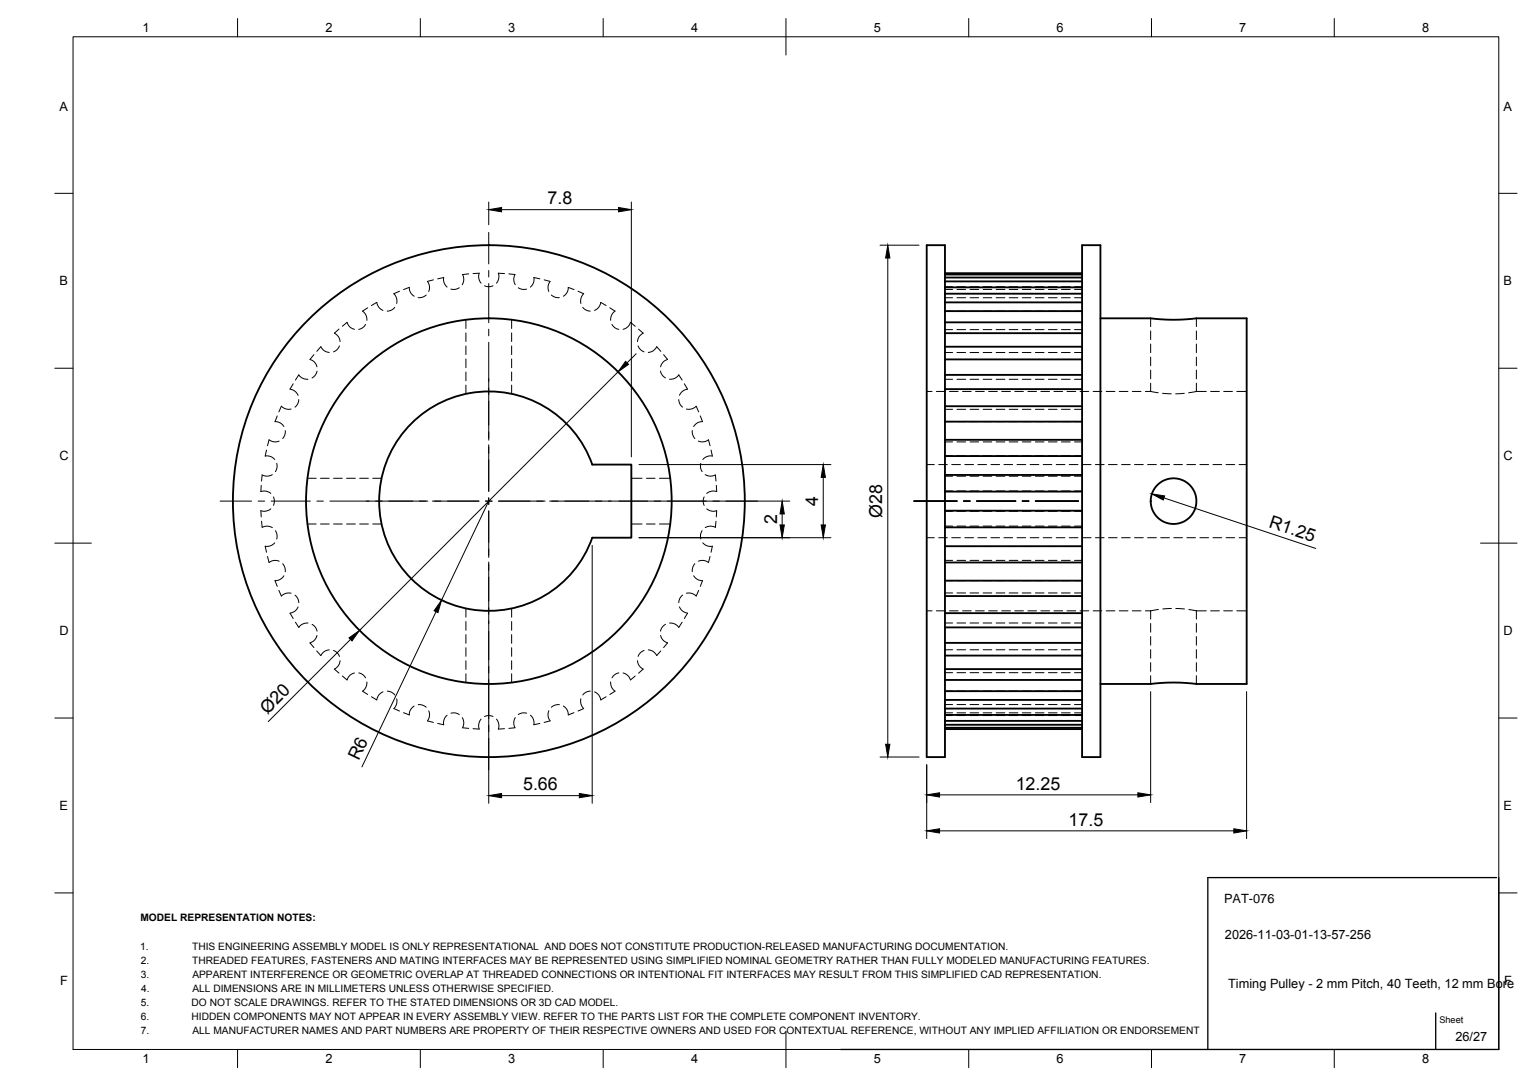
ISO-10303-21;
HEADER;
/* Generated by software containing ST-Developer
 * from STEP Tools, Inc. (www.steptools.com) 
 */

FILE_DESCRIPTION(
/* description */ ('Overhung pulley bearing cartridge'),
/* implementation_level */ '2;1');

FILE_NAME(
/* name */ 'Timing Pulley - 2 mm Pitch, 40 Teeth, 12 mm Bore.step',
/* time_stamp */ '2026-10-28T03:22:33-07:00',
/* author */ (''),
/* organization */ (''),
/* preprocessor_version */ 'ST-DEVELOPER v20.2',
/* originating_system */ 'Autodesk Translation Framework v15.17.0.0',
/* authorisation */ '');

FILE_SCHEMA (('AUTOMOTIVE_DESIGN { 1 0 10303 214 3 1 1 }'));
ENDSEC;

DATA;
#10=MECHANICAL_DESIGN_GEOMETRIC_PRESENTATION_REPRESENTATION('',(#310),#10963);
#189=B_SPLINE_CURVE_WITH_KNOTS('',3,(#10010,#10011,#10012,#10013,#10014,
#10015,#10016,#10017,#10018,#10019,#10020,#10021,#10022,#10023,#10024,#10025,
#10026,#10027),.UNSPECIFIED.,.F.,.F.,(4,2,2,2,2,2,2,2,4),(0.,0.0472365751919841,
0.0944731503839683,0.14170659898184,0.188940047579712,0.236173496177583,
0.283406944775455,0.330643519967439,0.377880095159423),.UNSPECIFIED.);
#190=B_SPLINE_CURVE_WITH_KNOTS('',3,(#10028,#10029,#10030,#10031,#10032,
#10033,#10034,#10035,#10036,#10037,#10038,#10039,#10040,#10041,#10042,#10043,
#10044,#10045),.UNSPECIFIED.,.F.,.F.,(4,2,2,2,2,2,2,2,4),(0.377880095159423,
0.425116670351408,0.472353245543392,0.519586694141263,0.566820142739135,
0.614053591337007,0.661287039934879,0.708523615126863,0.755760190318847),
 .UNSPECIFIED.);
#191=B_SPLINE_CURVE_WITH_KNOTS('',3,(#10048,#10049,#10050,#10051,#10052,
#10053,#10054,#10055,#10056,#10057,#10058,#10059,#10060,#10061,#10062,#10063,
#10064,#10065),.UNSPECIFIED.,.F.,.F.,(4,2,2,2,2,2,2,2,4),(0.,0.0472365751919841,
0.0944731503839682,0.14170659898184,0.188940047579712,0.236173496177583,
0.283406944775455,0.330643519967439,0.377880095159423),.UNSPECIFIED.);
#192=B_SPLINE_CURVE_WITH_KNOTS('',3,(#10066,#10067,#10068,#10069,#10070,
#10071,#10072,#10073,#10074,#10075,#10076,#10077,#10078,#10079,#10080,#10081,
#10082,#10083),.UNSPECIFIED.,.F.,.F.,(4,2,2,2,2,2,2,2,4),(0.377880095159423,
0.425116670351408,0.472353245543392,0.519586694141263,0.566820142739135,
0.614053591337007,0.661287039934879,0.708523615126863,0.755760190318847),
 .UNSPECIFIED.);
#193=B_SPLINE_CURVE_WITH_KNOTS('',3,(#10086,#10087,#10088,#10089,#10090,
#10091,#10092,#10093,#10094,#10095,#10096,#10097,#10098,#10099,#10100,#10101,
#10102,#10103),.UNSPECIFIED.,.F.,.F.,(4,2,2,2,2,2,2,2,4),(0.,0.0472365751919841,
0.0944731503839683,0.14170659898184,0.188940047579712,0.236173496177583,
0.283406944775455,0.330643519967439,0.377880095159423),.UNSPECIFIED.);
#194=B_SPLINE_CURVE_WITH_KNOTS('',3,(#10104,#10105,#10106,#10107,#10108,
#10109,#10110,#10111,#10112,#10113,#10114,#10115,#10116,#10117,#10118,#10119,
#10120,#10121),.UNSPECIFIED.,.F.,.F.,(4,2,2,2,2,2,2,2,4),(0.377880095159423,
0.425116670351408,0.472353245543392,0.519586694141263,0.566820142739135,
0.614053591337007,0.661287039934879,0.708523615126863,0.755760190318847),
 .UNSPECIFIED.);
#195=B_SPLINE_CURVE_WITH_KNOTS('',3,(#10125,#10126,#10127,#10128,#10129,
#10130,#10131,#10132,#10133,#10134),.UNSPECIFIED.,.F.,.F.,(4,2,2,2,4),(0.565665723963061,
0.61280433739166,0.659942950820258,0.70708195805217,0.754220965284082),
 .UNSPECIFIED.);
#196=B_SPLINE_CURVE_WITH_KNOTS('',3,(#10136,#10137,#10138,#10139,#10140,
#10141,#10142,#10143,#10144,#10145,#10146,#10147,#10148,#10149,#10150,#10151,
#10152,#10153),.UNSPECIFIED.,.F.,.F.,(4,2,2,2,2,2,2,2,4),(0.18855524132102,
0.235693854749619,0.282832468178217,0.329971475410129,0.377110482642041,
0.424249489873953,0.471388497105864,0.518527110534463,0.565665723963061),
 .UNSPECIFIED.);
#197=B_SPLINE_CURVE_WITH_KNOTS('',3,(#10154,#10155,#10156,#10157,#10158,
#10159,#10160,#10161,#10162,#10163),.UNSPECIFIED.,.F.,.F.,(4,2,2,2,4),(0.754220965284082,
0.801359972515993,0.848498979747905,0.895637593176504,0.942776206605102),
 .UNSPECIFIED.);
#198=B_SPLINE_CURVE_WITH_KNOTS('',3,(#10169,#10170,#10171,#10172,#10173,
#10174,#10175,#10176,#10177,#10178),.UNSPECIFIED.,.F.,.F.,(4,2,2,2,4),(0.565665723963061,
0.61280433739166,0.659942950820258,0.70708195805217,0.754220965284082),
 .UNSPECIFIED.);
#199=B_SPLINE_CURVE_WITH_KNOTS('',3,(#10180,#10181,#10182,#10183,#10184,
#10185,#10186,#10187,#10188,#10189,#10190,#10191,#10192,#10193,#10194,#10195,
#10196,#10197),.UNSPECIFIED.,.F.,.F.,(4,2,2,2,2,2,2,2,4),(0.18855524132102,
0.235693854749619,0.282832468178217,0.329971475410129,0.377110482642041,
0.424249489873953,0.471388497105864,0.518527110534463,0.565665723963061),
 .UNSPECIFIED.);
#200=B_SPLINE_CURVE_WITH_KNOTS('',3,(#10198,#10199,#10200,#10201,#10202,
#10203,#10204,#10205,#10206,#10207),.UNSPECIFIED.,.F.,.F.,(4,2,2,2,4),(0.754220965284082,
0.801359972515993,0.848498979747905,0.895637593176504,0.942776206605102),
 .UNSPECIFIED.);
#201=B_SPLINE_CURVE_WITH_KNOTS('',3,(#10217,#10218,#10219,#10220,#10221,
#10222,#10223,#10224,#10225,#10226,#10227,#10228,#10229,#10230,#10231,#10232,
#10233,#10234),.UNSPECIFIED.,.F.,.F.,(4,2,2,2,2,2,2,2,4),(0.18855524132102,
0.235693854749619,0.282832468178217,0.329971475410129,0.377110482642041,
0.424249489873953,0.471388497105864,0.518527110534463,0.565665723963061),
 .UNSPECIFIED.);
#202=B_SPLINE_CURVE_WITH_KNOTS('',3,(#10236,#10237,#10238,#10239,#10240,
#10241,#10242,#10243,#10244,#10245),.UNSPECIFIED.,.F.,.F.,(4,2,2,2,4),(0.565665723963061,
0.61280433739166,0.659942950820258,0.70708195805217,0.754220965284082),
 .UNSPECIFIED.);
#203=B_SPLINE_CURVE_WITH_KNOTS('',3,(#10246,#10247,#10248,#10249,#10250,
#10251,#10252,#10253,#10254,#10255),.UNSPECIFIED.,.F.,.F.,(4,2,2,2,4),(0.754220965284082,
0.801359972515993,0.848498979747905,0.895637593176504,0.942776206605102),
 .UNSPECIFIED.);
#204=B_SPLINE_CURVE_WITH_KNOTS('',3,(#10258,#10259,#10260,#10261,#10262,
#10263,#10264,#10265,#10266,#10267,#10268,#10269,#10270,#10271,#10272,#10273,
#10274,#10275),.UNSPECIFIED.,.F.,.F.,(4,2,2,2,2,2,2,2,4),(0.18855524132102,
0.235693854749619,0.282832468178217,0.329971475410129,0.377110482642041,
0.424249489873953,0.471388497105864,0.518527110534463,0.565665723963061),
 .UNSPECIFIED.);
#205=B_SPLINE_CURVE_WITH_KNOTS('',3,(#10277,#10278,#10279,#10280,#10281,
#10282,#10283,#10284,#10285,#10286),.UNSPECIFIED.,.F.,.F.,(4,2,2,2,4),(0.565665723963061,
0.61280433739166,0.659942950820258,0.70708195805217,0.754220965284082),
 .UNSPECIFIED.);
#206=B_SPLINE_CURVE_WITH_KNOTS('',3,(#10287,#10288,#10289,#10290,#10291,
#10292,#10293,#10294,#10295,#10296),.UNSPECIFIED.,.F.,.F.,(4,2,2,2,4),(0.754220965284082,
0.801359972515993,0.848498979747905,0.895637593176504,0.942776206605102),
 .UNSPECIFIED.);
#258=SHAPE_REPRESENTATION_RELATIONSHIP('SRR','None',#11080,#280);
#280=ADVANCED_BREP_SHAPE_REPRESENTATION('',(#338),#10960);
#310=STYLED_ITEM('',(#11246),#338);
#338=MANIFOLD_SOLID_BREP('Body1',#5679);
#421=FACE_BOUND('',#1199,.T.);
#422=FACE_BOUND('',#1202,.T.);
#423=FACE_BOUND('',#1204,.T.);
#424=FACE_BOUND('',#1205,.T.);
#425=FACE_BOUND('',#1206,.T.);
#426=FACE_BOUND('',#1210,.T.);
#427=FACE_BOUND('',#1211,.T.);
#428=FACE_BOUND('',#1212,.T.);
#429=FACE_BOUND('',#1216,.T.);
#430=FACE_BOUND('',#1218,.T.);
#431=FACE_BOUND('',#1221,.T.);
#432=FACE_BOUND('',#1223,.T.);
#550=PLANE('',#6385);
#551=PLANE('',#6386);
#552=PLANE('',#6388);
#553=PLANE('',#6389);
#554=PLANE('',#6401);
#555=PLANE('',#6402);
#556=PLANE('',#6486);
#557=PLANE('',#6487);
#788=FACE_OUTER_BOUND('',#1197,.T.);
#789=FACE_OUTER_BOUND('',#1198,.T.);
#790=FACE_OUTER_BOUND('',#1200,.T.);
#791=FACE_OUTER_BOUND('',#1201,.T.);
#792=FACE_OUTER_BOUND('',#1203,.T.);
#793=FACE_OUTER_BOUND('',#1207,.T.);
#794=FACE_OUTER_BOUND('',#1208,.T.);
#795=FACE_OUTER_BOUND('',#1209,.T.);
#796=FACE_OUTER_BOUND('',#1213,.T.);
#797=FACE_OUTER_BOUND('',#1214,.T.);
#798=FACE_OUTER_BOUND('',#1215,.T.);
#799=FACE_OUTER_BOUND('',#1217,.T.);
#800=FACE_OUTER_BOUND('',#1219,.T.);
#801=FACE_OUTER_BOUND('',#1220,.T.);
#802=FACE_OUTER_BOUND('',#1222,.T.);
#803=FACE_OUTER_BOUND('',#1224,.T.);
#804=FACE_OUTER_BOUND('',#1225,.T.);
#805=FACE_OUTER_BOUND('',#1226,.T.);
#806=FACE_OUTER_BOUND('',#1227,.T.);
#807=FACE_OUTER_BOUND('',#1228,.T.);
#808=FACE_OUTER_BOUND('',#1229,.T.);
#809=FACE_OUTER_BOUND('',#1230,.T.);
#810=FACE_OUTER_BOUND('',#1231,.T.);
#811=FACE_OUTER_BOUND('',#1232,.T.);
#812=FACE_OUTER_BOUND('',#1233,.T.);
#813=FACE_OUTER_BOUND('',#1234,.T.);
#814=FACE_OUTER_BOUND('',#1235,.T.);
#815=FACE_OUTER_BOUND('',#1236,.T.);
#816=FACE_OUTER_BOUND('',#1237,.T.);
#817=FACE_OUTER_BOUND('',#1238,.T.);
#818=FACE_OUTER_BOUND('',#1239,.T.);
#819=FACE_OUTER_BOUND('',#1240,.T.);
#820=FACE_OUTER_BOUND('',#1241,.T.);
#821=FACE_OUTER_BOUND('',#1242,.T.);
#822=FACE_OUTER_BOUND('',#1243,.T.);
#823=FACE_OUTER_BOUND('',#1244,.T.);
#824=FACE_OUTER_BOUND('',#1245,.T.);
#825=FACE_OUTER_BOUND('',#1246,.T.);
#826=FACE_OUTER_BOUND('',#1247,.T.);
#827=FACE_OUTER_BOUND('',#1248,.T.);
#828=FACE_OUTER_BOUND('',#1249,.T.);
#829=FACE_OUTER_BOUND('',#1250,.T.);
#830=FACE_OUTER_BOUND('',#1251,.T.);
#831=FACE_OUTER_BOUND('',#1252,.T.);
#832=FACE_OUTER_BOUND('',#1253,.T.);
#833=FACE_OUTER_BOUND('',#1254,.T.);
#834=FACE_OUTER_BOUND('',#1255,.T.);
#835=FACE_OUTER_BOUND('',#1256,.T.);
#836=FACE_OUTER_BOUND('',#1257,.T.);
#837=FACE_OUTER_BOUND('',#1258,.T.);
#838=FACE_OUTER_BOUND('',#1259,.T.);
#839=FACE_OUTER_BOUND('',#1260,.T.);
#840=FACE_OUTER_BOUND('',#1261,.T.);
#841=FACE_OUTER_BOUND('',#1262,.T.);
#842=FACE_OUTER_BOUND('',#1263,.T.);
#843=FACE_OUTER_BOUND('',#1264,.T.);
#844=FACE_OUTER_BOUND('',#1265,.T.);
#845=FACE_OUTER_BOUND('',#1266,.T.);
#846=FACE_OUTER_BOUND('',#1267,.T.);
#847=FACE_OUTER_BOUND('',#1268,.T.);
#848=FACE_OUTER_BOUND('',#1269,.T.);
#849=FACE_OUTER_BOUND('',#1270,.T.);
#850=FACE_OUTER_BOUND('',#1271,.T.);
#851=FACE_OUTER_BOUND('',#1272,.T.);
#852=FACE_OUTER_BOUND('',#1273,.T.);
#853=FACE_OUTER_BOUND('',#1274,.T.);
#854=FACE_OUTER_BOUND('',#1275,.T.);
#855=FACE_OUTER_BOUND('',#1276,.T.);
#856=FACE_OUTER_BOUND('',#1277,.T.);
#857=FACE_OUTER_BOUND('',#1278,.T.);
#858=FACE_OUTER_BOUND('',#1279,.T.);
#859=FACE_OUTER_BOUND('',#1280,.T.);
#860=FACE_OUTER_BOUND('',#1281,.T.);
#861=FACE_OUTER_BOUND('',#1282,.T.);
#862=FACE_OUTER_BOUND('',#1283,.T.);
#863=FACE_OUTER_BOUND('',#1284,.T.);
#864=FACE_OUTER_BOUND('',#1285,.T.);
#865=FACE_OUTER_BOUND('',#1286,.T.);
#866=FACE_OUTER_BOUND('',#1287,.T.);
#867=FACE_OUTER_BOUND('',#1288,.T.);
#868=FACE_OUTER_BOUND('',#1289,.T.);
#869=FACE_OUTER_BOUND('',#1290,.T.);
#870=FACE_OUTER_BOUND('',#1291,.T.);
#871=FACE_OUTER_BOUND('',#1292,.T.);
#872=FACE_OUTER_BOUND('',#1293,.T.);
#873=FACE_OUTER_BOUND('',#1294,.T.);
#874=FACE_OUTER_BOUND('',#1295,.T.);
#875=FACE_OUTER_BOUND('',#1296,.T.);
#876=FACE_OUTER_BOUND('',#1297,.T.);
#877=FACE_OUTER_BOUND('',#1298,.T.);
#878=FACE_OUTER_BOUND('',#1299,.T.);
#879=FACE_OUTER_BOUND('',#1300,.T.);
#880=FACE_OUTER_BOUND('',#1301,.T.);
#881=FACE_OUTER_BOUND('',#1302,.T.);
#882=FACE_OUTER_BOUND('',#1303,.T.);
#883=FACE_OUTER_BOUND('',#1304,.T.);
#1197=EDGE_LOOP('',(#4499,#4500,#4501,#4502));
#1198=EDGE_LOOP('',(#4503,#4504,#4505,#4506));
#1199=EDGE_LOOP('',(#4507));
#1200=EDGE_LOOP('',(#4508,#4509,#4510,#4511));
#1201=EDGE_LOOP('',(#4512));
#1202=EDGE_LOOP('',(#4513,#4514,#4515,#4516));
#1203=EDGE_LOOP('',(#4517,#4518,#4519,#4520));
#1204=EDGE_LOOP('',(#4521,#4522));
#1205=EDGE_LOOP('',(#4523,#4524));
#1206=EDGE_LOOP('',(#4525,#4526));
#1207=EDGE_LOOP('',(#4527,#4528,#4529,#4530,#4531,#4532,#4533));
#1208=EDGE_LOOP('',(#4534,#4535,#4536,#4537,#4538,#4539,#4540));
#1209=EDGE_LOOP('',(#4541,#4542,#4543,#4544,#4545,#4546,#4547,#4548,#4549));
#1210=EDGE_LOOP('',(#4550,#4551,#4552));
#1211=EDGE_LOOP('',(#4553,#4554,#4555));
#1212=EDGE_LOOP('',(#4556,#4557,#4558));
#1213=EDGE_LOOP('',(#4559,#4560,#4561,#4562,#4563,#4564));
#1214=EDGE_LOOP('',(#4565,#4566,#4567,#4568,#4569,#4570,#4571));
#1215=EDGE_LOOP('',(#4572));
#1216=EDGE_LOOP('',(#4573,#4574,#4575,#4576));
#1217=EDGE_LOOP('',(#4577));
#1218=EDGE_LOOP('',(#4578,#4579,#4580,#4581,#4582,#4583,#4584,#4585,#4586,
#4587,#4588,#4589,#4590,#4591,#4592,#4593,#4594,#4595,#4596,#4597,#4598,
#4599,#4600,#4601,#4602,#4603,#4604,#4605,#4606,#4607,#4608,#4609,#4610,
#4611,#4612,#4613,#4614,#4615,#4616,#4617,#4618,#4619,#4620,#4621,#4622,
#4623,#4624,#4625,#4626,#4627,#4628,#4629,#4630,#4631,#4632,#4633,#4634,
#4635,#4636,#4637,#4638,#4639,#4640,#4641,#4642,#4643,#4644,#4645,#4646,
#4647,#4648,#4649,#4650,#4651,#4652,#4653,#4654,#4655,#4656,#4657));
#1219=EDGE_LOOP('',(#4658,#4659,#4660,#4661));
#1220=EDGE_LOOP('',(#4662));
#1221=EDGE_LOOP('',(#4663));
#1222=EDGE_LOOP('',(#4664));
#1223=EDGE_LOOP('',(#4665,#4666,#4667,#4668,#4669,#4670,#4671,#4672,#4673,
#4674,#4675,#4676,#4677,#4678,#4679,#4680,#4681,#4682,#4683,#4684,#4685,
#4686,#4687,#4688,#4689,#4690,#4691,#4692,#4693,#4694,#4695,#4696,#4697,
#4698,#4699,#4700,#4701,#4702,#4703,#4704,#4705,#4706,#4707,#4708,#4709,
#4710,#4711,#4712,#4713,#4714,#4715,#4716,#4717,#4718,#4719,#4720,#4721,
#4722,#4723,#4724,#4725,#4726,#4727,#4728,#4729,#4730,#4731,#4732,#4733,
#4734,#4735,#4736,#4737,#4738,#4739,#4740,#4741,#4742,#4743,#4744));
#1224=EDGE_LOOP('',(#4745,#4746,#4747,#4748));
#1225=EDGE_LOOP('',(#4749,#4750,#4751,#4752));
#1226=EDGE_LOOP('',(#4753,#4754,#4755,#4756));
#1227=EDGE_LOOP('',(#4757,#4758,#4759,#4760));
#1228=EDGE_LOOP('',(#4761,#4762,#4763,#4764));
#1229=EDGE_LOOP('',(#4765,#4766,#4767,#4768));
#1230=EDGE_LOOP('',(#4769,#4770,#4771,#4772));
#1231=EDGE_LOOP('',(#4773,#4774,#4775,#4776));
#1232=EDGE_LOOP('',(#4777,#4778,#4779,#4780));
#1233=EDGE_LOOP('',(#4781,#4782,#4783,#4784));
#1234=EDGE_LOOP('',(#4785,#4786,#4787,#4788));
#1235=EDGE_LOOP('',(#4789,#4790,#4791,#4792));
#1236=EDGE_LOOP('',(#4793,#4794,#4795,#4796));
#1237=EDGE_LOOP('',(#4797,#4798,#4799,#4800));
#1238=EDGE_LOOP('',(#4801,#4802,#4803,#4804));
#1239=EDGE_LOOP('',(#4805,#4806,#4807,#4808));
#1240=EDGE_LOOP('',(#4809,#4810,#4811,#4812));
#1241=EDGE_LOOP('',(#4813,#4814,#4815,#4816));
#1242=EDGE_LOOP('',(#4817,#4818,#4819,#4820));
#1243=EDGE_LOOP('',(#4821,#4822,#4823,#4824));
#1244=EDGE_LOOP('',(#4825,#4826,#4827,#4828));
#1245=EDGE_LOOP('',(#4829,#4830,#4831,#4832));
#1246=EDGE_LOOP('',(#4833,#4834,#4835,#4836));
#1247=EDGE_LOOP('',(#4837,#4838,#4839,#4840));
#1248=EDGE_LOOP('',(#4841,#4842,#4843,#4844));
#1249=EDGE_LOOP('',(#4845,#4846,#4847,#4848));
#1250=EDGE_LOOP('',(#4849,#4850,#4851,#4852));
#1251=EDGE_LOOP('',(#4853,#4854,#4855,#4856));
#1252=EDGE_LOOP('',(#4857,#4858,#4859,#4860));
#1253=EDGE_LOOP('',(#4861,#4862,#4863,#4864));
#1254=EDGE_LOOP('',(#4865,#4866,#4867,#4868));
#1255=EDGE_LOOP('',(#4869,#4870,#4871,#4872));
#1256=EDGE_LOOP('',(#4873,#4874,#4875,#4876));
#1257=EDGE_LOOP('',(#4877,#4878,#4879,#4880));
#1258=EDGE_LOOP('',(#4881,#4882,#4883,#4884));
#1259=EDGE_LOOP('',(#4885,#4886,#4887,#4888));
#1260=EDGE_LOOP('',(#4889,#4890,#4891,#4892));
#1261=EDGE_LOOP('',(#4893,#4894,#4895,#4896));
#1262=EDGE_LOOP('',(#4897,#4898,#4899,#4900));
#1263=EDGE_LOOP('',(#4901,#4902,#4903,#4904));
#1264=EDGE_LOOP('',(#4905,#4906,#4907,#4908));
#1265=EDGE_LOOP('',(#4909,#4910,#4911,#4912));
#1266=EDGE_LOOP('',(#4913,#4914,#4915,#4916));
#1267=EDGE_LOOP('',(#4917,#4918,#4919,#4920));
#1268=EDGE_LOOP('',(#4921,#4922,#4923,#4924));
#1269=EDGE_LOOP('',(#4925,#4926,#4927,#4928));
#1270=EDGE_LOOP('',(#4929,#4930,#4931,#4932));
#1271=EDGE_LOOP('',(#4933,#4934,#4935,#4936));
#1272=EDGE_LOOP('',(#4937,#4938,#4939,#4940));
#1273=EDGE_LOOP('',(#4941,#4942,#4943,#4944));
#1274=EDGE_LOOP('',(#4945,#4946,#4947,#4948));
#1275=EDGE_LOOP('',(#4949,#4950,#4951,#4952));
#1276=EDGE_LOOP('',(#4953,#4954,#4955,#4956));
#1277=EDGE_LOOP('',(#4957,#4958,#4959,#4960));
#1278=EDGE_LOOP('',(#4961,#4962,#4963,#4964));
#1279=EDGE_LOOP('',(#4965,#4966,#4967,#4968));
#1280=EDGE_LOOP('',(#4969,#4970,#4971,#4972));
#1281=EDGE_LOOP('',(#4973,#4974,#4975,#4976));
#1282=EDGE_LOOP('',(#4977,#4978,#4979,#4980));
#1283=EDGE_LOOP('',(#4981,#4982,#4983,#4984));
#1284=EDGE_LOOP('',(#4985,#4986,#4987,#4988));
#1285=EDGE_LOOP('',(#4989,#4990,#4991,#4992));
#1286=EDGE_LOOP('',(#4993,#4994,#4995,#4996));
#1287=EDGE_LOOP('',(#4997,#4998,#4999,#5000));
#1288=EDGE_LOOP('',(#5001,#5002,#5003,#5004));
#1289=EDGE_LOOP('',(#5005,#5006,#5007,#5008));
#1290=EDGE_LOOP('',(#5009,#5010,#5011,#5012));
#1291=EDGE_LOOP('',(#5013,#5014,#5015,#5016));
#1292=EDGE_LOOP('',(#5017,#5018,#5019,#5020));
#1293=EDGE_LOOP('',(#5021,#5022,#5023,#5024));
#1294=EDGE_LOOP('',(#5025,#5026,#5027,#5028));
#1295=EDGE_LOOP('',(#5029,#5030,#5031,#5032));
#1296=EDGE_LOOP('',(#5033,#5034,#5035,#5036));
#1297=EDGE_LOOP('',(#5037,#5038,#5039,#5040));
#1298=EDGE_LOOP('',(#5041,#5042,#5043,#5044));
#1299=EDGE_LOOP('',(#5045,#5046,#5047,#5048));
#1300=EDGE_LOOP('',(#5049,#5050,#5051,#5052));
#1301=EDGE_LOOP('',(#5053,#5054,#5055,#5056));
#1302=EDGE_LOOP('',(#5057,#5058,#5059,#5060));
#1303=EDGE_LOOP('',(#5061,#5062,#5063,#5064));
#1304=EDGE_LOOP('',(#5065,#5066,#5067,#5068));
#1527=LINE('',#9982,#1869);
#1528=LINE('',#9984,#1870);
#1529=LINE('',#9986,#1871);
#1530=LINE('',#9987,#1872);
#1531=LINE('',#9990,#1873);
#1532=LINE('',#9992,#1874);
#1533=LINE('',#9993,#1875);
#1534=LINE('',#9998,#1876);
#1535=LINE('',#10000,#1877);
#1536=LINE('',#10001,#1878);
#1537=LINE('',#10164,#1879);
#1538=LINE('',#10167,#1880);
#1539=LINE('',#10211,#1881);
#1540=LINE('',#10213,#1882);
#1541=LINE('',#10298,#1883);
#1542=LINE('',#10300,#1884);
#1543=LINE('',#10468,#1885);
#1544=LINE('',#10634,#1886);
#1545=LINE('',#10636,#1887);
#1546=LINE('',#10637,#1888);
#1547=LINE('',#10639,#1889);
#1548=LINE('',#10641,#1890);
#1549=LINE('',#10643,#1891);
#1550=LINE('',#10645,#1892);
#1551=LINE('',#10647,#1893);
#1552=LINE('',#10649,#1894);
#1553=LINE('',#10651,#1895);
#1554=LINE('',#10653,#1896);
#1555=LINE('',#10655,#1897);
#1556=LINE('',#10657,#1898);
#1557=LINE('',#10659,#1899);
#1558=LINE('',#10661,#1900);
#1559=LINE('',#10663,#1901);
#1560=LINE('',#10665,#1902);
#1561=LINE('',#10667,#1903);
#1562=LINE('',#10669,#1904);
#1563=LINE('',#10671,#1905);
#1564=LINE('',#10673,#1906);
#1565=LINE('',#10675,#1907);
#1566=LINE('',#10677,#1908);
#1567=LINE('',#10679,#1909);
#1568=LINE('',#10681,#1910);
#1569=LINE('',#10683,#1911);
#1570=LINE('',#10685,#1912);
#1571=LINE('',#10687,#1913);
#1572=LINE('',#10689,#1914);
#1573=LINE('',#10691,#1915);
#1574=LINE('',#10693,#1916);
#1575=LINE('',#10695,#1917);
#1576=LINE('',#10697,#1918);
#1577=LINE('',#10699,#1919);
#1578=LINE('',#10701,#1920);
#1579=LINE('',#10703,#1921);
#1580=LINE('',#10705,#1922);
#1581=LINE('',#10707,#1923);
#1582=LINE('',#10709,#1924);
#1583=LINE('',#10711,#1925);
#1584=LINE('',#10713,#1926);
#1585=LINE('',#10715,#1927);
#1586=LINE('',#10717,#1928);
#1587=LINE('',#10719,#1929);
#1588=LINE('',#10721,#1930);
#1589=LINE('',#10723,#1931);
#1590=LINE('',#10725,#1932);
#1591=LINE('',#10727,#1933);
#1592=LINE('',#10729,#1934);
#1593=LINE('',#10731,#1935);
#1594=LINE('',#10733,#1936);
#1595=LINE('',#10735,#1937);
#1596=LINE('',#10737,#1938);
#1597=LINE('',#10739,#1939);
#1598=LINE('',#10741,#1940);
#1599=LINE('',#10743,#1941);
#1600=LINE('',#10745,#1942);
#1601=LINE('',#10747,#1943);
#1602=LINE('',#10749,#1944);
#1603=LINE('',#10751,#1945);
#1604=LINE('',#10753,#1946);
#1605=LINE('',#10755,#1947);
#1606=LINE('',#10757,#1948);
#1607=LINE('',#10759,#1949);
#1608=LINE('',#10761,#1950);
#1609=LINE('',#10763,#1951);
#1610=LINE('',#10765,#1952);
#1611=LINE('',#10767,#1953);
#1612=LINE('',#10769,#1954);
#1613=LINE('',#10771,#1955);
#1614=LINE('',#10773,#1956);
#1615=LINE('',#10775,#1957);
#1616=LINE('',#10777,#1958);
#1617=LINE('',#10779,#1959);
#1618=LINE('',#10781,#1960);
#1619=LINE('',#10783,#1961);
#1620=LINE('',#10785,#1962);
#1621=LINE('',#10787,#1963);
#1622=LINE('',#10789,#1964);
#1623=LINE('',#10791,#1965);
#1624=LINE('',#10793,#1966);
#1869=VECTOR('',#7809,1.);
#1870=VECTOR('',#7810,1.);
#1871=VECTOR('',#7811,1.);
#1872=VECTOR('',#7812,1.);
#1873=VECTOR('',#7815,1.);
#1874=VECTOR('',#7816,1.);
#1875=VECTOR('',#7817,1.);
#1876=VECTOR('',#7822,1.);
#1877=VECTOR('',#7823,1.);
#1878=VECTOR('',#7824,1.);
#1879=VECTOR('',#7837,0.125);
#1880=VECTOR('',#7840,0.125);
#1881=VECTOR('',#7845,1.);
#1882=VECTOR('',#7846,1.);
#1883=VECTOR('',#7851,0.125);
#1884=VECTOR('',#7854,0.125);
#1885=VECTOR('',#8025,1.4);
#1886=VECTOR('',#8194,1.4);
#1887=VECTOR('',#8197,1.);
#1888=VECTOR('',#8198,1.);
#1889=VECTOR('',#8201,1.);
#1890=VECTOR('',#8204,1.);
#1891=VECTOR('',#8207,1.);
#1892=VECTOR('',#8210,1.);
#1893=VECTOR('',#8213,1.);
#1894=VECTOR('',#8216,1.);
#1895=VECTOR('',#8219,1.);
#1896=VECTOR('',#8222,1.);
#1897=VECTOR('',#8225,1.);
#1898=VECTOR('',#8228,1.);
#1899=VECTOR('',#8231,1.);
#1900=VECTOR('',#8234,1.);
#1901=VECTOR('',#8237,1.);
#1902=VECTOR('',#8240,1.);
#1903=VECTOR('',#8243,1.);
#1904=VECTOR('',#8246,1.);
#1905=VECTOR('',#8249,1.);
#1906=VECTOR('',#8252,1.);
#1907=VECTOR('',#8255,1.);
#1908=VECTOR('',#8258,1.);
#1909=VECTOR('',#8261,1.);
#1910=VECTOR('',#8264,1.);
#1911=VECTOR('',#8267,1.);
#1912=VECTOR('',#8270,1.);
#1913=VECTOR('',#8273,1.);
#1914=VECTOR('',#8276,1.);
#1915=VECTOR('',#8279,1.);
#1916=VECTOR('',#8282,1.);
#1917=VECTOR('',#8285,1.);
#1918=VECTOR('',#8288,1.);
#1919=VECTOR('',#8291,1.);
#1920=VECTOR('',#8294,1.);
#1921=VECTOR('',#8297,1.);
#1922=VECTOR('',#8300,1.);
#1923=VECTOR('',#8303,1.);
#1924=VECTOR('',#8306,1.);
#1925=VECTOR('',#8309,1.);
#1926=VECTOR('',#8312,1.);
#1927=VECTOR('',#8315,1.);
#1928=VECTOR('',#8318,1.);
#1929=VECTOR('',#8321,1.);
#1930=VECTOR('',#8324,1.);
#1931=VECTOR('',#8327,1.);
#1932=VECTOR('',#8330,1.);
#1933=VECTOR('',#8333,1.);
#1934=VECTOR('',#8336,1.);
#1935=VECTOR('',#8339,1.);
#1936=VECTOR('',#8342,1.);
#1937=VECTOR('',#8345,1.);
#1938=VECTOR('',#8348,1.);
#1939=VECTOR('',#8351,1.);
#1940=VECTOR('',#8354,1.);
#1941=VECTOR('',#8357,1.);
#1942=VECTOR('',#8360,1.);
#1943=VECTOR('',#8363,1.);
#1944=VECTOR('',#8366,1.);
#1945=VECTOR('',#8369,1.);
#1946=VECTOR('',#8372,1.);
#1947=VECTOR('',#8375,1.);
#1948=VECTOR('',#8378,1.);
#1949=VECTOR('',#8381,1.);
#1950=VECTOR('',#8384,1.);
#1951=VECTOR('',#8387,1.);
#1952=VECTOR('',#8390,1.);
#1953=VECTOR('',#8393,1.);
#1954=VECTOR('',#8396,1.);
#1955=VECTOR('',#8399,1.);
#1956=VECTOR('',#8402,1.);
#1957=VECTOR('',#8405,1.);
#1958=VECTOR('',#8408,1.);
#1959=VECTOR('',#8411,1.);
#1960=VECTOR('',#8414,1.);
#1961=VECTOR('',#8417,1.);
#1962=VECTOR('',#8420,1.);
#1963=VECTOR('',#8423,1.);
#1964=VECTOR('',#8426,1.);
#1965=VECTOR('',#8429,1.);
#1966=VECTOR('',#8432,1.);
#2210=CIRCLE('',#6387,0.125);
#2211=CIRCLE('',#6390,1.4);
#2212=CIRCLE('',#6391,0.6);
#2213=CIRCLE('',#6393,0.6);
#2214=CIRCLE('',#6397,1.);
#2215=CIRCLE('',#6398,1.);
#2216=CIRCLE('',#6403,1.4);
#2217=CIRCLE('',#6404,0.0555000000000001);
#2218=CIRCLE('',#6405,1.24783954473516);
#2219=CIRCLE('',#6406,0.0555000000000001);
#2220=CIRCLE('',#6407,1.24783954473516);
#2221=CIRCLE('',#6408,0.0555000000000001);
#2222=CIRCLE('',#6409,1.24783954473516);
#2223=CIRCLE('',#6410,0.0555000000000001);
#2224=CIRCLE('',#6411,1.24783954473516);
#2225=CIRCLE('',#6412,0.0555000000000001);
#2226=CIRCLE('',#6413,1.24783954473516);
#2227=CIRCLE('',#6414,0.0555000000000001);
#2228=CIRCLE('',#6415,1.24783954473516);
#2229=CIRCLE('',#6416,0.0555000000000001);
#2230=CIRCLE('',#6417,1.24783954473516);
#2231=CIRCLE('',#6418,0.0555000000000001);
#2232=CIRCLE('',#6419,1.24783954473516);
#2233=CIRCLE('',#6420,0.0555000000000001);
#2234=CIRCLE('',#6421,1.24783954473516);
#2235=CIRCLE('',#6422,0.0555000000000001);
#2236=CIRCLE('',#6423,1.24783954473516);
#2237=CIRCLE('',#6424,0.0555000000000001);
#2238=CIRCLE('',#6425,1.24783954473516);
#2239=CIRCLE('',#6426,0.0555000000000001);
#2240=CIRCLE('',#6427,1.24783954473516);
#2241=CIRCLE('',#6428,0.0555000000000001);
#2242=CIRCLE('',#6429,1.24783954473516);
#2243=CIRCLE('',#6430,0.0555000000000001);
#2244=CIRCLE('',#6431,1.24783954473516);
#2245=CIRCLE('',#6432,0.0555000000000001);
#2246=CIRCLE('',#6433,1.24783954473516);
#2247=CIRCLE('',#6434,0.0555000000000001);
#2248=CIRCLE('',#6435,1.24783954473516);
#2249=CIRCLE('',#6436,0.0555000000000001);
#2250=CIRCLE('',#6437,1.24783954473516);
#2251=CIRCLE('',#6438,0.0555000000000001);
#2252=CIRCLE('',#6439,1.24783954473516);
#2253=CIRCLE('',#6440,0.0555000000000001);
#2254=CIRCLE('',#6441,1.24783954473516);
#2255=CIRCLE('',#6442,0.0555000000000001);
#2256=CIRCLE('',#6443,1.24783954473516);
#2257=CIRCLE('',#6444,0.0555000000000001);
#2258=CIRCLE('',#6445,1.24783954473516);
#2259=CIRCLE('',#6446,0.0555000000000001);
#2260=CIRCLE('',#6447,1.24783954473516);
#2261=CIRCLE('',#6448,0.0555000000000001);
#2262=CIRCLE('',#6449,1.24783954473516);
#2263=CIRCLE('',#6450,0.0555000000000001);
#2264=CIRCLE('',#6451,1.24783954473516);
#2265=CIRCLE('',#6452,0.0555000000000001);
#2266=CIRCLE('',#6453,1.24783954473516);
#2267=CIRCLE('',#6454,0.0555000000000001);
#2268=CIRCLE('',#6455,1.24783954473516);
#2269=CIRCLE('',#6456,0.0555000000000001);
#2270=CIRCLE('',#6457,1.24783954473516);
#2271=CIRCLE('',#6458,0.0555000000000001);
#2272=CIRCLE('',#6459,1.24783954473516);
#2273=CIRCLE('',#6460,0.0555000000000001);
#2274=CIRCLE('',#6461,1.24783954473516);
#2275=CIRCLE('',#6462,0.0555000000000001);
#2276=CIRCLE('',#6463,1.24783954473516);
#2277=CIRCLE('',#6464,0.0555000000000001);
#2278=CIRCLE('',#6465,1.24783954473516);
#2279=CIRCLE('',#6466,0.0555000000000001);
#2280=CIRCLE('',#6467,1.24783954473516);
#2281=CIRCLE('',#6468,0.0555000000000001);
#2282=CIRCLE('',#6469,1.24783954473516);
#2283=CIRCLE('',#6470,0.0555000000000001);
#2284=CIRCLE('',#6471,1.24783954473516);
#2285=CIRCLE('',#6472,0.0555000000000001);
#2286=CIRCLE('',#6473,1.24783954473516);
#2287=CIRCLE('',#6474,0.0555000000000001);
#2288=CIRCLE('',#6475,1.24783954473516);
#2289=CIRCLE('',#6476,0.0555000000000001);
#2290=CIRCLE('',#6477,1.24783954473516);
#2291=CIRCLE('',#6478,0.0555000000000001);
#2292=CIRCLE('',#6479,1.24783954473516);
#2293=CIRCLE('',#6480,0.0555000000000001);
#2294=CIRCLE('',#6481,1.24783954473516);
#2295=CIRCLE('',#6482,0.0555000000000001);
#2296=CIRCLE('',#6483,1.24783954473516);
#2297=CIRCLE('',#6485,1.4);
#2298=CIRCLE('',#6488,1.4);
#2299=CIRCLE('',#6489,0.0555000000000001);
#2300=CIRCLE('',#6490,1.24783954473516);
#2301=CIRCLE('',#6491,0.0555000000000001);
#2302=CIRCLE('',#6492,1.24783954473516);
#2303=CIRCLE('',#6493,0.0555000000000001);
#2304=CIRCLE('',#6494,1.24783954473516);
#2305=CIRCLE('',#6495,0.0555000000000001);
#2306=CIRCLE('',#6496,1.24783954473516);
#2307=CIRCLE('',#6497,0.0555000000000001);
#2308=CIRCLE('',#6498,1.24783954473516);
#2309=CIRCLE('',#6499,0.0555000000000001);
#2310=CIRCLE('',#6500,1.24783954473516);
#2311=CIRCLE('',#6501,0.0555000000000001);
#2312=CIRCLE('',#6502,1.24783954473516);
#2313=CIRCLE('',#6503,0.0555000000000001);
#2314=CIRCLE('',#6504,1.24783954473516);
#2315=CIRCLE('',#6505,0.0555000000000001);
#2316=CIRCLE('',#6506,1.24783954473516);
#2317=CIRCLE('',#6507,0.0555000000000001);
#2318=CIRCLE('',#6508,1.24783954473516);
#2319=CIRCLE('',#6509,0.0555000000000001);
#2320=CIRCLE('',#6510,1.24783954473516);
#2321=CIRCLE('',#6511,0.0555000000000001);
#2322=CIRCLE('',#6512,1.24783954473516);
#2323=CIRCLE('',#6513,0.0555000000000001);
#2324=CIRCLE('',#6514,1.24783954473516);
#2325=CIRCLE('',#6515,0.0555000000000001);
#2326=CIRCLE('',#6516,1.24783954473516);
#2327=CIRCLE('',#6517,0.0555000000000001);
#2328=CIRCLE('',#6518,1.24783954473516);
#2329=CIRCLE('',#6519,0.0555000000000001);
#2330=CIRCLE('',#6520,1.24783954473516);
#2331=CIRCLE('',#6521,0.0555000000000001);
#2332=CIRCLE('',#6522,1.24783954473516);
#2333=CIRCLE('',#6523,0.0555000000000001);
#2334=CIRCLE('',#6524,1.24783954473516);
#2335=CIRCLE('',#6525,0.0555000000000001);
#2336=CIRCLE('',#6526,1.24783954473516);
#2337=CIRCLE('',#6527,0.0555000000000001);
#2338=CIRCLE('',#6528,1.24783954473516);
#2339=CIRCLE('',#6529,0.0555000000000001);
#2340=CIRCLE('',#6530,1.24783954473516);
#2341=CIRCLE('',#6531,0.0555000000000001);
#2342=CIRCLE('',#6532,1.24783954473516);
#2343=CIRCLE('',#6533,0.0555000000000001);
#2344=CIRCLE('',#6534,1.24783954473516);
#2345=CIRCLE('',#6535,0.0555000000000001);
#2346=CIRCLE('',#6536,1.24783954473516);
#2347=CIRCLE('',#6537,0.0555000000000001);
#2348=CIRCLE('',#6538,1.24783954473516);
#2349=CIRCLE('',#6539,0.0555000000000001);
#2350=CIRCLE('',#6540,1.24783954473516);
#2351=CIRCLE('',#6541,0.0555000000000001);
#2352=CIRCLE('',#6542,1.24783954473516);
#2353=CIRCLE('',#6543,0.0555000000000001);
#2354=CIRCLE('',#6544,1.24783954473516);
#2355=CIRCLE('',#6545,0.0555000000000001);
#2356=CIRCLE('',#6546,1.24783954473516);
#2357=CIRCLE('',#6547,0.0555000000000001);
#2358=CIRCLE('',#6548,1.24783954473516);
#2359=CIRCLE('',#6549,0.0555000000000001);
#2360=CIRCLE('',#6550,1.24783954473516);
#2361=CIRCLE('',#6551,0.0555000000000001);
#2362=CIRCLE('',#6552,1.24783954473516);
#2363=CIRCLE('',#6553,0.0555000000000001);
#2364=CIRCLE('',#6554,1.24783954473516);
#2365=CIRCLE('',#6555,0.0555000000000001);
#2366=CIRCLE('',#6556,1.24783954473516);
#2367=CIRCLE('',#6557,0.0555000000000001);
#2368=CIRCLE('',#6558,1.24783954473516);
#2369=CIRCLE('',#6559,0.0555000000000001);
#2370=CIRCLE('',#6560,1.24783954473516);
#2371=CIRCLE('',#6561,0.0555000000000001);
#2372=CIRCLE('',#6562,1.24783954473516);
#2373=CIRCLE('',#6563,0.0555000000000001);
#2374=CIRCLE('',#6564,1.24783954473516);
#2375=CIRCLE('',#6565,0.0555000000000001);
#2376=CIRCLE('',#6566,1.24783954473516);
#2377=CIRCLE('',#6567,0.0555000000000001);
#2378=CIRCLE('',#6568,1.24783954473516);
#2671=VERTEX_POINT('',#9980);
#2672=VERTEX_POINT('',#9981);
#2673=VERTEX_POINT('',#9983);
#2674=VERTEX_POINT('',#9985);
#2675=VERTEX_POINT('',#9989);
#2676=VERTEX_POINT('',#9991);
#2677=VERTEX_POINT('',#9994);
#2678=VERTEX_POINT('',#9997);
#2679=VERTEX_POINT('',#9999);
#2680=VERTEX_POINT('',#10003);
#2681=VERTEX_POINT('',#10008);
#2682=VERTEX_POINT('',#10009);
#2683=VERTEX_POINT('',#10046);
#2684=VERTEX_POINT('',#10047);
#2685=VERTEX_POINT('',#10084);
#2686=VERTEX_POINT('',#10085);
#2687=VERTEX_POINT('',#10123);
#2688=VERTEX_POINT('',#10124);
#2689=VERTEX_POINT('',#10135);
#2690=VERTEX_POINT('',#10166);
#2691=VERTEX_POINT('',#10168);
#2692=VERTEX_POINT('',#10179);
#2693=VERTEX_POINT('',#10209);
#2694=VERTEX_POINT('',#10212);
#2695=VERTEX_POINT('',#10215);
#2696=VERTEX_POINT('',#10216);
#2697=VERTEX_POINT('',#10235);
#2698=VERTEX_POINT('',#10256);
#2699=VERTEX_POINT('',#10257);
#2700=VERTEX_POINT('',#10276);
#2701=VERTEX_POINT('',#10303);
#2702=VERTEX_POINT('',#10305);
#2703=VERTEX_POINT('',#10306);
#2704=VERTEX_POINT('',#10308);
#2705=VERTEX_POINT('',#10310);
#2706=VERTEX_POINT('',#10312);
#2707=VERTEX_POINT('',#10314);
#2708=VERTEX_POINT('',#10316);
#2709=VERTEX_POINT('',#10318);
#2710=VERTEX_POINT('',#10320);
#2711=VERTEX_POINT('',#10322);
#2712=VERTEX_POINT('',#10324);
#2713=VERTEX_POINT('',#10326);
#2714=VERTEX_POINT('',#10328);
#2715=VERTEX_POINT('',#10330);
#2716=VERTEX_POINT('',#10332);
#2717=VERTEX_POINT('',#10334);
#2718=VERTEX_POINT('',#10336);
#2719=VERTEX_POINT('',#10338);
#2720=VERTEX_POINT('',#10340);
#2721=VERTEX_POINT('',#10342);
#2722=VERTEX_POINT('',#10344);
#2723=VERTEX_POINT('',#10346);
#2724=VERTEX_POINT('',#10348);
#2725=VERTEX_POINT('',#10350);
#2726=VERTEX_POINT('',#10352);
#2727=VERTEX_POINT('',#10354);
#2728=VERTEX_POINT('',#10356);
#2729=VERTEX_POINT('',#10358);
#2730=VERTEX_POINT('',#10360);
#2731=VERTEX_POINT('',#10362);
#2732=VERTEX_POINT('',#10364);
#2733=VERTEX_POINT('',#10366);
#2734=VERTEX_POINT('',#10368);
#2735=VERTEX_POINT('',#10370);
#2736=VERTEX_POINT('',#10372);
#2737=VERTEX_POINT('',#10374);
#2738=VERTEX_POINT('',#10376);
#2739=VERTEX_POINT('',#10378);
#2740=VERTEX_POINT('',#10380);
#2741=VERTEX_POINT('',#10382);
#2742=VERTEX_POINT('',#10384);
#2743=VERTEX_POINT('',#10386);
#2744=VERTEX_POINT('',#10388);
#2745=VERTEX_POINT('',#10390);
#2746=VERTEX_POINT('',#10392);
#2747=VERTEX_POINT('',#10394);
#2748=VERTEX_POINT('',#10396);
#2749=VERTEX_POINT('',#10398);
#2750=VERTEX_POINT('',#10400);
#2751=VERTEX_POINT('',#10402);
#2752=VERTEX_POINT('',#10404);
#2753=VERTEX_POINT('',#10406);
#2754=VERTEX_POINT('',#10408);
#2755=VERTEX_POINT('',#10410);
#2756=VERTEX_POINT('',#10412);
#2757=VERTEX_POINT('',#10414);
#2758=VERTEX_POINT('',#10416);
#2759=VERTEX_POINT('',#10418);
#2760=VERTEX_POINT('',#10420);
#2761=VERTEX_POINT('',#10422);
#2762=VERTEX_POINT('',#10424);
#2763=VERTEX_POINT('',#10426);
#2764=VERTEX_POINT('',#10428);
#2765=VERTEX_POINT('',#10430);
#2766=VERTEX_POINT('',#10432);
#2767=VERTEX_POINT('',#10434);
#2768=VERTEX_POINT('',#10436);
#2769=VERTEX_POINT('',#10438);
#2770=VERTEX_POINT('',#10440);
#2771=VERTEX_POINT('',#10442);
#2772=VERTEX_POINT('',#10444);
#2773=VERTEX_POINT('',#10446);
#2774=VERTEX_POINT('',#10448);
#2775=VERTEX_POINT('',#10450);
#2776=VERTEX_POINT('',#10452);
#2777=VERTEX_POINT('',#10454);
#2778=VERTEX_POINT('',#10456);
#2779=VERTEX_POINT('',#10458);
#2780=VERTEX_POINT('',#10460);
#2781=VERTEX_POINT('',#10462);
#2782=VERTEX_POINT('',#10466);
#2783=VERTEX_POINT('',#10471);
#2784=VERTEX_POINT('',#10473);
#2785=VERTEX_POINT('',#10474);
#2786=VERTEX_POINT('',#10476);
#2787=VERTEX_POINT('',#10478);
#2788=VERTEX_POINT('',#10480);
#2789=VERTEX_POINT('',#10482);
#2790=VERTEX_POINT('',#10484);
#2791=VERTEX_POINT('',#10486);
#2792=VERTEX_POINT('',#10488);
#2793=VERTEX_POINT('',#10490);
#2794=VERTEX_POINT('',#10492);
#2795=VERTEX_POINT('',#10494);
#2796=VERTEX_POINT('',#10496);
#2797=VERTEX_POINT('',#10498);
#2798=VERTEX_POINT('',#10500);
#2799=VERTEX_POINT('',#10502);
#2800=VERTEX_POINT('',#10504);
#2801=VERTEX_POINT('',#10506);
#2802=VERTEX_POINT('',#10508);
#2803=VERTEX_POINT('',#10510);
#2804=VERTEX_POINT('',#10512);
#2805=VERTEX_POINT('',#10514);
#2806=VERTEX_POINT('',#10516);
#2807=VERTEX_POINT('',#10518);
#2808=VERTEX_POINT('',#10520);
#2809=VERTEX_POINT('',#10522);
#2810=VERTEX_POINT('',#10524);
#2811=VERTEX_POINT('',#10526);
#2812=VERTEX_POINT('',#10528);
#2813=VERTEX_POINT('',#10530);
#2814=VERTEX_POINT('',#10532);
#2815=VERTEX_POINT('',#10534);
#2816=VERTEX_POINT('',#10536);
#2817=VERTEX_POINT('',#10538);
#2818=VERTEX_POINT('',#10540);
#2819=VERTEX_POINT('',#10542);
#2820=VERTEX_POINT('',#10544);
#2821=VERTEX_POINT('',#10546);
#2822=VERTEX_POINT('',#10548);
#2823=VERTEX_POINT('',#10550);
#2824=VERTEX_POINT('',#10552);
#2825=VERTEX_POINT('',#10554);
#2826=VERTEX_POINT('',#10556);
#2827=VERTEX_POINT('',#10558);
#2828=VERTEX_POINT('',#10560);
#2829=VERTEX_POINT('',#10562);
#2830=VERTEX_POINT('',#10564);
#2831=VERTEX_POINT('',#10566);
#2832=VERTEX_POINT('',#10568);
#2833=VERTEX_POINT('',#10570);
#2834=VERTEX_POINT('',#10572);
#2835=VERTEX_POINT('',#10574);
#2836=VERTEX_POINT('',#10576);
#2837=VERTEX_POINT('',#10578);
#2838=VERTEX_POINT('',#10580);
#2839=VERTEX_POINT('',#10582);
#2840=VERTEX_POINT('',#10584);
#2841=VERTEX_POINT('',#10586);
#2842=VERTEX_POINT('',#10588);
#2843=VERTEX_POINT('',#10590);
#2844=VERTEX_POINT('',#10592);
#2845=VERTEX_POINT('',#10594);
#2846=VERTEX_POINT('',#10596);
#2847=VERTEX_POINT('',#10598);
#2848=VERTEX_POINT('',#10600);
#2849=VERTEX_POINT('',#10602);
#2850=VERTEX_POINT('',#10604);
#2851=VERTEX_POINT('',#10606);
#2852=VERTEX_POINT('',#10608);
#2853=VERTEX_POINT('',#10610);
#2854=VERTEX_POINT('',#10612);
#2855=VERTEX_POINT('',#10614);
#2856=VERTEX_POINT('',#10616);
#2857=VERTEX_POINT('',#10618);
#2858=VERTEX_POINT('',#10620);
#2859=VERTEX_POINT('',#10622);
#2860=VERTEX_POINT('',#10624);
#2861=VERTEX_POINT('',#10626);
#2862=VERTEX_POINT('',#10628);
#2863=VERTEX_POINT('',#10630);
#3319=EDGE_CURVE('',#2671,#2672,#1527,.T.);
#3320=EDGE_CURVE('',#2671,#2673,#1528,.T.);
#3321=EDGE_CURVE('',#2674,#2673,#1529,.T.);
#3322=EDGE_CURVE('',#2672,#2674,#1530,.T.);
#3323=EDGE_CURVE('',#2675,#2671,#1531,.T.);
#3324=EDGE_CURVE('',#2675,#2676,#1532,.T.);
#3325=EDGE_CURVE('',#2673,#2676,#1533,.T.);
#3326=EDGE_CURVE('',#2677,#2677,#2210,.T.);
#3327=EDGE_CURVE('',#2678,#2675,#1534,.T.);
#3328=EDGE_CURVE('',#2679,#2678,#1535,.T.);
#3329=EDGE_CURVE('',#2676,#2679,#1536,.T.);
#3330=EDGE_CURVE('',#2680,#2680,#2211,.T.);
#3331=EDGE_CURVE('',#2679,#2674,#2212,.T.);
#3332=EDGE_CURVE('',#2672,#2678,#2213,.T.);
#3333=EDGE_CURVE('',#2681,#2682,#189,.T.);
#3334=EDGE_CURVE('',#2682,#2681,#190,.T.);
#3335=EDGE_CURVE('',#2683,#2684,#191,.T.);
#3336=EDGE_CURVE('',#2684,#2683,#192,.T.);
#3337=EDGE_CURVE('',#2685,#2686,#193,.T.);
#3338=EDGE_CURVE('',#2686,#2685,#194,.T.);
#3339=EDGE_CURVE('',#2687,#2688,#195,.T.);
#3340=EDGE_CURVE('',#2689,#2687,#196,.T.);
#3341=EDGE_CURVE('',#2688,#2689,#197,.T.);
#3342=EDGE_CURVE('',#2688,#2684,#1537,.T.);
#3343=EDGE_CURVE('',#2686,#2690,#1538,.T.);
#3344=EDGE_CURVE('',#2691,#2690,#198,.T.);
#3345=EDGE_CURVE('',#2692,#2691,#199,.T.);
#3346=EDGE_CURVE('',#2690,#2692,#200,.T.);
#3347=EDGE_CURVE('',#2693,#2693,#2214,.T.);
#3348=EDGE_CURVE('',#2693,#2689,#1539,.T.);
#3349=EDGE_CURVE('',#2687,#2694,#1540,.T.);
#3350=EDGE_CURVE('',#2694,#2694,#2215,.T.);
#3351=EDGE_CURVE('',#2695,#2696,#201,.T.);
#3352=EDGE_CURVE('',#2696,#2697,#202,.T.);
#3353=EDGE_CURVE('',#2697,#2695,#203,.T.);
#3354=EDGE_CURVE('',#2698,#2699,#204,.T.);
#3355=EDGE_CURVE('',#2699,#2700,#205,.T.);
#3356=EDGE_CURVE('',#2700,#2698,#206,.T.);
#3357=EDGE_CURVE('',#2697,#2677,#1541,.T.);
#3358=EDGE_CURVE('',#2682,#2700,#1542,.T.);
#3359=EDGE_CURVE('',#2701,#2701,#2216,.T.);
#3360=EDGE_CURVE('',#2702,#2703,#2217,.T.);
#3361=EDGE_CURVE('',#2704,#2703,#2218,.T.);
#3362=EDGE_CURVE('',#2704,#2705,#2219,.T.);
#3363=EDGE_CURVE('',#2706,#2705,#2220,.T.);
#3364=EDGE_CURVE('',#2706,#2707,#2221,.T.);
#3365=EDGE_CURVE('',#2708,#2707,#2222,.T.);
#3366=EDGE_CURVE('',#2708,#2709,#2223,.T.);
#3367=EDGE_CURVE('',#2710,#2709,#2224,.T.);
#3368=EDGE_CURVE('',#2710,#2711,#2225,.T.);
#3369=EDGE_CURVE('',#2712,#2711,#2226,.T.);
#3370=EDGE_CURVE('',#2712,#2713,#2227,.T.);
#3371=EDGE_CURVE('',#2714,#2713,#2228,.T.);
#3372=EDGE_CURVE('',#2714,#2715,#2229,.T.);
#3373=EDGE_CURVE('',#2716,#2715,#2230,.T.);
#3374=EDGE_CURVE('',#2716,#2717,#2231,.T.);
#3375=EDGE_CURVE('',#2718,#2717,#2232,.T.);
#3376=EDGE_CURVE('',#2718,#2719,#2233,.T.);
#3377=EDGE_CURVE('',#2720,#2719,#2234,.T.);
#3378=EDGE_CURVE('',#2720,#2721,#2235,.T.);
#3379=EDGE_CURVE('',#2722,#2721,#2236,.T.);
#3380=EDGE_CURVE('',#2722,#2723,#2237,.T.);
#3381=EDGE_CURVE('',#2724,#2723,#2238,.T.);
#3382=EDGE_CURVE('',#2724,#2725,#2239,.T.);
#3383=EDGE_CURVE('',#2726,#2725,#2240,.T.);
#3384=EDGE_CURVE('',#2726,#2727,#2241,.T.);
#3385=EDGE_CURVE('',#2728,#2727,#2242,.T.);
#3386=EDGE_CURVE('',#2728,#2729,#2243,.T.);
#3387=EDGE_CURVE('',#2730,#2729,#2244,.T.);
#3388=EDGE_CURVE('',#2730,#2731,#2245,.T.);
#3389=EDGE_CURVE('',#2732,#2731,#2246,.T.);
#3390=EDGE_CURVE('',#2732,#2733,#2247,.T.);
#3391=EDGE_CURVE('',#2734,#2733,#2248,.T.);
#3392=EDGE_CURVE('',#2734,#2735,#2249,.T.);
#3393=EDGE_CURVE('',#2736,#2735,#2250,.T.);
#3394=EDGE_CURVE('',#2736,#2737,#2251,.T.);
#3395=EDGE_CURVE('',#2738,#2737,#2252,.T.);
#3396=EDGE_CURVE('',#2738,#2739,#2253,.T.);
#3397=EDGE_CURVE('',#2740,#2739,#2254,.T.);
#3398=EDGE_CURVE('',#2740,#2741,#2255,.T.);
#3399=EDGE_CURVE('',#2742,#2741,#2256,.T.);
#3400=EDGE_CURVE('',#2742,#2743,#2257,.T.);
#3401=EDGE_CURVE('',#2744,#2743,#2258,.T.);
#3402=EDGE_CURVE('',#2744,#2745,#2259,.T.);
#3403=EDGE_CURVE('',#2746,#2745,#2260,.T.);
#3404=EDGE_CURVE('',#2746,#2747,#2261,.T.);
#3405=EDGE_CURVE('',#2748,#2747,#2262,.T.);
#3406=EDGE_CURVE('',#2748,#2749,#2263,.T.);
#3407=EDGE_CURVE('',#2750,#2749,#2264,.T.);
#3408=EDGE_CURVE('',#2750,#2751,#2265,.T.);
#3409=EDGE_CURVE('',#2752,#2751,#2266,.T.);
#3410=EDGE_CURVE('',#2752,#2753,#2267,.T.);
#3411=EDGE_CURVE('',#2754,#2753,#2268,.T.);
#3412=EDGE_CURVE('',#2754,#2755,#2269,.T.);
#3413=EDGE_CURVE('',#2756,#2755,#2270,.T.);
#3414=EDGE_CURVE('',#2756,#2757,#2271,.T.);
#3415=EDGE_CURVE('',#2758,#2757,#2272,.T.);
#3416=EDGE_CURVE('',#2758,#2759,#2273,.T.);
#3417=EDGE_CURVE('',#2760,#2759,#2274,.T.);
#3418=EDGE_CURVE('',#2760,#2761,#2275,.T.);
#3419=EDGE_CURVE('',#2762,#2761,#2276,.T.);
#3420=EDGE_CURVE('',#2762,#2763,#2277,.T.);
#3421=EDGE_CURVE('',#2764,#2763,#2278,.T.);
#3422=EDGE_CURVE('',#2764,#2765,#2279,.T.);
#3423=EDGE_CURVE('',#2766,#2765,#2280,.T.);
#3424=EDGE_CURVE('',#2766,#2767,#2281,.T.);
#3425=EDGE_CURVE('',#2768,#2767,#2282,.T.);
#3426=EDGE_CURVE('',#2768,#2769,#2283,.T.);
#3427=EDGE_CURVE('',#2770,#2769,#2284,.T.);
#3428=EDGE_CURVE('',#2770,#2771,#2285,.T.);
#3429=EDGE_CURVE('',#2772,#2771,#2286,.T.);
#3430=EDGE_CURVE('',#2772,#2773,#2287,.T.);
#3431=EDGE_CURVE('',#2774,#2773,#2288,.T.);
#3432=EDGE_CURVE('',#2774,#2775,#2289,.T.);
#3433=EDGE_CURVE('',#2776,#2775,#2290,.T.);
#3434=EDGE_CURVE('',#2776,#2777,#2291,.T.);
#3435=EDGE_CURVE('',#2778,#2777,#2292,.T.);
#3436=EDGE_CURVE('',#2778,#2779,#2293,.T.);
#3437=EDGE_CURVE('',#2780,#2779,#2294,.T.);
#3438=EDGE_CURVE('',#2780,#2781,#2295,.T.);
#3439=EDGE_CURVE('',#2702,#2781,#2296,.T.);
#3440=EDGE_CURVE('',#2782,#2782,#2297,.T.);
#3441=EDGE_CURVE('',#2782,#2701,#1543,.T.);
#3442=EDGE_CURVE('',#2783,#2783,#2298,.T.);
#3443=EDGE_CURVE('',#2784,#2785,#2299,.T.);
#3444=EDGE_CURVE('',#2785,#2786,#2300,.T.);
#3445=EDGE_CURVE('',#2786,#2787,#2301,.T.);
#3446=EDGE_CURVE('',#2787,#2788,#2302,.T.);
#3447=EDGE_CURVE('',#2788,#2789,#2303,.T.);
#3448=EDGE_CURVE('',#2789,#2790,#2304,.T.);
#3449=EDGE_CURVE('',#2790,#2791,#2305,.T.);
#3450=EDGE_CURVE('',#2791,#2792,#2306,.T.);
#3451=EDGE_CURVE('',#2792,#2793,#2307,.T.);
#3452=EDGE_CURVE('',#2793,#2794,#2308,.T.);
#3453=EDGE_CURVE('',#2794,#2795,#2309,.T.);
#3454=EDGE_CURVE('',#2795,#2796,#2310,.T.);
#3455=EDGE_CURVE('',#2796,#2797,#2311,.T.);
#3456=EDGE_CURVE('',#2797,#2798,#2312,.T.);
#3457=EDGE_CURVE('',#2798,#2799,#2313,.T.);
#3458=EDGE_CURVE('',#2799,#2800,#2314,.T.);
#3459=EDGE_CURVE('',#2800,#2801,#2315,.T.);
#3460=EDGE_CURVE('',#2801,#2802,#2316,.T.);
#3461=EDGE_CURVE('',#2802,#2803,#2317,.T.);
#3462=EDGE_CURVE('',#2803,#2804,#2318,.T.);
#3463=EDGE_CURVE('',#2804,#2805,#2319,.T.);
#3464=EDGE_CURVE('',#2805,#2806,#2320,.T.);
#3465=EDGE_CURVE('',#2806,#2807,#2321,.T.);
#3466=EDGE_CURVE('',#2807,#2808,#2322,.T.);
#3467=EDGE_CURVE('',#2808,#2809,#2323,.T.);
#3468=EDGE_CURVE('',#2809,#2810,#2324,.T.);
#3469=EDGE_CURVE('',#2810,#2811,#2325,.T.);
#3470=EDGE_CURVE('',#2811,#2812,#2326,.T.);
#3471=EDGE_CURVE('',#2812,#2813,#2327,.T.);
#3472=EDGE_CURVE('',#2813,#2814,#2328,.T.);
#3473=EDGE_CURVE('',#2814,#2815,#2329,.T.);
#3474=EDGE_CURVE('',#2815,#2816,#2330,.T.);
#3475=EDGE_CURVE('',#2816,#2817,#2331,.T.);
#3476=EDGE_CURVE('',#2817,#2818,#2332,.T.);
#3477=EDGE_CURVE('',#2818,#2819,#2333,.T.);
#3478=EDGE_CURVE('',#2819,#2820,#2334,.T.);
#3479=EDGE_CURVE('',#2820,#2821,#2335,.T.);
#3480=EDGE_CURVE('',#2821,#2822,#2336,.T.);
#3481=EDGE_CURVE('',#2822,#2823,#2337,.T.);
#3482=EDGE_CURVE('',#2823,#2824,#2338,.T.);
#3483=EDGE_CURVE('',#2824,#2825,#2339,.T.);
#3484=EDGE_CURVE('',#2825,#2826,#2340,.T.);
#3485=EDGE_CURVE('',#2826,#2827,#2341,.T.);
#3486=EDGE_CURVE('',#2827,#2828,#2342,.T.);
#3487=EDGE_CURVE('',#2828,#2829,#2343,.T.);
#3488=EDGE_CURVE('',#2829,#2830,#2344,.T.);
#3489=EDGE_CURVE('',#2830,#2831,#2345,.T.);
#3490=EDGE_CURVE('',#2831,#2832,#2346,.T.);
#3491=EDGE_CURVE('',#2832,#2833,#2347,.T.);
#3492=EDGE_CURVE('',#2833,#2834,#2348,.T.);
#3493=EDGE_CURVE('',#2834,#2835,#2349,.T.);
#3494=EDGE_CURVE('',#2835,#2836,#2350,.T.);
#3495=EDGE_CURVE('',#2836,#2837,#2351,.T.);
#3496=EDGE_CURVE('',#2837,#2838,#2352,.T.);
#3497=EDGE_CURVE('',#2838,#2839,#2353,.T.);
#3498=EDGE_CURVE('',#2839,#2840,#2354,.T.);
#3499=EDGE_CURVE('',#2840,#2841,#2355,.T.);
#3500=EDGE_CURVE('',#2841,#2842,#2356,.T.);
#3501=EDGE_CURVE('',#2842,#2843,#2357,.T.);
#3502=EDGE_CURVE('',#2843,#2844,#2358,.T.);
#3503=EDGE_CURVE('',#2844,#2845,#2359,.T.);
#3504=EDGE_CURVE('',#2845,#2846,#2360,.T.);
#3505=EDGE_CURVE('',#2846,#2847,#2361,.T.);
#3506=EDGE_CURVE('',#2847,#2848,#2362,.T.);
#3507=EDGE_CURVE('',#2848,#2849,#2363,.T.);
#3508=EDGE_CURVE('',#2849,#2850,#2364,.T.);
#3509=EDGE_CURVE('',#2850,#2851,#2365,.T.);
#3510=EDGE_CURVE('',#2851,#2852,#2366,.T.);
#3511=EDGE_CURVE('',#2852,#2853,#2367,.T.);
#3512=EDGE_CURVE('',#2853,#2854,#2368,.T.);
#3513=EDGE_CURVE('',#2854,#2855,#2369,.T.);
#3514=EDGE_CURVE('',#2855,#2856,#2370,.T.);
#3515=EDGE_CURVE('',#2856,#2857,#2371,.T.);
#3516=EDGE_CURVE('',#2857,#2858,#2372,.T.);
#3517=EDGE_CURVE('',#2858,#2859,#2373,.T.);
#3518=EDGE_CURVE('',#2859,#2860,#2374,.T.);
#3519=EDGE_CURVE('',#2860,#2861,#2375,.T.);
#3520=EDGE_CURVE('',#2861,#2862,#2376,.T.);
#3521=EDGE_CURVE('',#2862,#2863,#2377,.T.);
#3522=EDGE_CURVE('',#2863,#2784,#2378,.T.);
#3523=EDGE_CURVE('',#2680,#2783,#1544,.T.);
#3524=EDGE_CURVE('',#2785,#2702,#1545,.T.);
#3525=EDGE_CURVE('',#2703,#2784,#1546,.T.);
#3526=EDGE_CURVE('',#2863,#2704,#1547,.T.);
#3527=EDGE_CURVE('',#2705,#2862,#1548,.T.);
#3528=EDGE_CURVE('',#2861,#2706,#1549,.T.);
#3529=EDGE_CURVE('',#2707,#2860,#1550,.T.);
#3530=EDGE_CURVE('',#2859,#2708,#1551,.T.);
#3531=EDGE_CURVE('',#2709,#2858,#1552,.T.);
#3532=EDGE_CURVE('',#2857,#2710,#1553,.T.);
#3533=EDGE_CURVE('',#2711,#2856,#1554,.T.);
#3534=EDGE_CURVE('',#2855,#2712,#1555,.T.);
#3535=EDGE_CURVE('',#2713,#2854,#1556,.T.);
#3536=EDGE_CURVE('',#2853,#2714,#1557,.T.);
#3537=EDGE_CURVE('',#2715,#2852,#1558,.T.);
#3538=EDGE_CURVE('',#2851,#2716,#1559,.T.);
#3539=EDGE_CURVE('',#2717,#2850,#1560,.T.);
#3540=EDGE_CURVE('',#2849,#2718,#1561,.T.);
#3541=EDGE_CURVE('',#2719,#2848,#1562,.T.);
#3542=EDGE_CURVE('',#2847,#2720,#1563,.T.);
#3543=EDGE_CURVE('',#2721,#2846,#1564,.T.);
#3544=EDGE_CURVE('',#2845,#2722,#1565,.T.);
#3545=EDGE_CURVE('',#2723,#2844,#1566,.T.);
#3546=EDGE_CURVE('',#2843,#2724,#1567,.T.);
#3547=EDGE_CURVE('',#2725,#2842,#1568,.T.);
#3548=EDGE_CURVE('',#2841,#2726,#1569,.T.);
#3549=EDGE_CURVE('',#2727,#2840,#1570,.T.);
#3550=EDGE_CURVE('',#2839,#2728,#1571,.T.);
#3551=EDGE_CURVE('',#2729,#2838,#1572,.T.);
#3552=EDGE_CURVE('',#2837,#2730,#1573,.T.);
#3553=EDGE_CURVE('',#2731,#2836,#1574,.T.);
#3554=EDGE_CURVE('',#2835,#2732,#1575,.T.);
#3555=EDGE_CURVE('',#2733,#2834,#1576,.T.);
#3556=EDGE_CURVE('',#2833,#2734,#1577,.T.);
#3557=EDGE_CURVE('',#2735,#2832,#1578,.T.);
#3558=EDGE_CURVE('',#2831,#2736,#1579,.T.);
#3559=EDGE_CURVE('',#2737,#2830,#1580,.T.);
#3560=EDGE_CURVE('',#2829,#2738,#1581,.T.);
#3561=EDGE_CURVE('',#2739,#2828,#1582,.T.);
#3562=EDGE_CURVE('',#2827,#2740,#1583,.T.);
#3563=EDGE_CURVE('',#2741,#2826,#1584,.T.);
#3564=EDGE_CURVE('',#2825,#2742,#1585,.T.);
#3565=EDGE_CURVE('',#2743,#2824,#1586,.T.);
#3566=EDGE_CURVE('',#2823,#2744,#1587,.T.);
#3567=EDGE_CURVE('',#2745,#2822,#1588,.T.);
#3568=EDGE_CURVE('',#2821,#2746,#1589,.T.);
#3569=EDGE_CURVE('',#2747,#2820,#1590,.T.);
#3570=EDGE_CURVE('',#2819,#2748,#1591,.T.);
#3571=EDGE_CURVE('',#2749,#2818,#1592,.T.);
#3572=EDGE_CURVE('',#2817,#2750,#1593,.T.);
#3573=EDGE_CURVE('',#2751,#2816,#1594,.T.);
#3574=EDGE_CURVE('',#2815,#2752,#1595,.T.);
#3575=EDGE_CURVE('',#2753,#2814,#1596,.T.);
#3576=EDGE_CURVE('',#2813,#2754,#1597,.T.);
#3577=EDGE_CURVE('',#2755,#2812,#1598,.T.);
#3578=EDGE_CURVE('',#2811,#2756,#1599,.T.);
#3579=EDGE_CURVE('',#2757,#2810,#1600,.T.);
#3580=EDGE_CURVE('',#2809,#2758,#1601,.T.);
#3581=EDGE_CURVE('',#2759,#2808,#1602,.T.);
#3582=EDGE_CURVE('',#2807,#2760,#1603,.T.);
#3583=EDGE_CURVE('',#2761,#2806,#1604,.T.);
#3584=EDGE_CURVE('',#2805,#2762,#1605,.T.);
#3585=EDGE_CURVE('',#2763,#2804,#1606,.T.);
#3586=EDGE_CURVE('',#2803,#2764,#1607,.T.);
#3587=EDGE_CURVE('',#2765,#2802,#1608,.T.);
#3588=EDGE_CURVE('',#2801,#2766,#1609,.T.);
#3589=EDGE_CURVE('',#2767,#2800,#1610,.T.);
#3590=EDGE_CURVE('',#2799,#2768,#1611,.T.);
#3591=EDGE_CURVE('',#2769,#2798,#1612,.T.);
#3592=EDGE_CURVE('',#2797,#2770,#1613,.T.);
#3593=EDGE_CURVE('',#2771,#2796,#1614,.T.);
#3594=EDGE_CURVE('',#2795,#2772,#1615,.T.);
#3595=EDGE_CURVE('',#2773,#2794,#1616,.T.);
#3596=EDGE_CURVE('',#2793,#2774,#1617,.T.);
#3597=EDGE_CURVE('',#2775,#2792,#1618,.T.);
#3598=EDGE_CURVE('',#2791,#2776,#1619,.T.);
#3599=EDGE_CURVE('',#2777,#2790,#1620,.T.);
#3600=EDGE_CURVE('',#2789,#2778,#1621,.T.);
#3601=EDGE_CURVE('',#2779,#2788,#1622,.T.);
#3602=EDGE_CURVE('',#2781,#2786,#1623,.T.);
#3603=EDGE_CURVE('',#2787,#2780,#1624,.T.);
#4499=ORIENTED_EDGE('',*,*,#3319,.F.);
#4500=ORIENTED_EDGE('',*,*,#3320,.T.);
#4501=ORIENTED_EDGE('',*,*,#3321,.F.);
#4502=ORIENTED_EDGE('',*,*,#3322,.F.);
#4503=ORIENTED_EDGE('',*,*,#3323,.F.);
#4504=ORIENTED_EDGE('',*,*,#3324,.T.);
#4505=ORIENTED_EDGE('',*,*,#3325,.F.);
#4506=ORIENTED_EDGE('',*,*,#3320,.F.);
#4507=ORIENTED_EDGE('',*,*,#3326,.F.);
#4508=ORIENTED_EDGE('',*,*,#3327,.F.);
#4509=ORIENTED_EDGE('',*,*,#3328,.F.);
#4510=ORIENTED_EDGE('',*,*,#3329,.F.);
#4511=ORIENTED_EDGE('',*,*,#3324,.F.);
#4512=ORIENTED_EDGE('',*,*,#3330,.T.);
#4513=ORIENTED_EDGE('',*,*,#3321,.T.);
#4514=ORIENTED_EDGE('',*,*,#3325,.T.);
#4515=ORIENTED_EDGE('',*,*,#3329,.T.);
#4516=ORIENTED_EDGE('',*,*,#3331,.T.);
#4517=ORIENTED_EDGE('',*,*,#3322,.T.);
#4518=ORIENTED_EDGE('',*,*,#3331,.F.);
#4519=ORIENTED_EDGE('',*,*,#3328,.T.);
#4520=ORIENTED_EDGE('',*,*,#3332,.F.);
#4521=ORIENTED_EDGE('',*,*,#3333,.T.);
#4522=ORIENTED_EDGE('',*,*,#3334,.T.);
#4523=ORIENTED_EDGE('',*,*,#3335,.T.);
#4524=ORIENTED_EDGE('',*,*,#3336,.T.);
#4525=ORIENTED_EDGE('',*,*,#3337,.T.);
#4526=ORIENTED_EDGE('',*,*,#3338,.T.);
#4527=ORIENTED_EDGE('',*,*,#3339,.F.);
#4528=ORIENTED_EDGE('',*,*,#3340,.F.);
#4529=ORIENTED_EDGE('',*,*,#3341,.F.);
#4530=ORIENTED_EDGE('',*,*,#3342,.T.);
#4531=ORIENTED_EDGE('',*,*,#3335,.F.);
#4532=ORIENTED_EDGE('',*,*,#3336,.F.);
#4533=ORIENTED_EDGE('',*,*,#3342,.F.);
#4534=ORIENTED_EDGE('',*,*,#3337,.F.);
#4535=ORIENTED_EDGE('',*,*,#3338,.F.);
#4536=ORIENTED_EDGE('',*,*,#3343,.T.);
#4537=ORIENTED_EDGE('',*,*,#3344,.F.);
#4538=ORIENTED_EDGE('',*,*,#3345,.F.);
#4539=ORIENTED_EDGE('',*,*,#3346,.F.);
#4540=ORIENTED_EDGE('',*,*,#3343,.F.);
#4541=ORIENTED_EDGE('',*,*,#3347,.F.);
#4542=ORIENTED_EDGE('',*,*,#3348,.T.);
#4543=ORIENTED_EDGE('',*,*,#3340,.T.);
#4544=ORIENTED_EDGE('',*,*,#3349,.T.);
#4545=ORIENTED_EDGE('',*,*,#3350,.F.);
#4546=ORIENTED_EDGE('',*,*,#3349,.F.);
#4547=ORIENTED_EDGE('',*,*,#3339,.T.);
#4548=ORIENTED_EDGE('',*,*,#3341,.T.);
#4549=ORIENTED_EDGE('',*,*,#3348,.F.);
#4550=ORIENTED_EDGE('',*,*,#3345,.T.);
#4551=ORIENTED_EDGE('',*,*,#3344,.T.);
#4552=ORIENTED_EDGE('',*,*,#3346,.T.);
#4553=ORIENTED_EDGE('',*,*,#3351,.T.);
#4554=ORIENTED_EDGE('',*,*,#3352,.T.);
#4555=ORIENTED_EDGE('',*,*,#3353,.T.);
#4556=ORIENTED_EDGE('',*,*,#3354,.T.);
#4557=ORIENTED_EDGE('',*,*,#3355,.T.);
#4558=ORIENTED_EDGE('',*,*,#3356,.T.);
#4559=ORIENTED_EDGE('',*,*,#3352,.F.);
#4560=ORIENTED_EDGE('',*,*,#3351,.F.);
#4561=ORIENTED_EDGE('',*,*,#3353,.F.);
#4562=ORIENTED_EDGE('',*,*,#3357,.T.);
#4563=ORIENTED_EDGE('',*,*,#3326,.T.);
#4564=ORIENTED_EDGE('',*,*,#3357,.F.);
#4565=ORIENTED_EDGE('',*,*,#3333,.F.);
#4566=ORIENTED_EDGE('',*,*,#3334,.F.);
#4567=ORIENTED_EDGE('',*,*,#3358,.T.);
#4568=ORIENTED_EDGE('',*,*,#3355,.F.);
#4569=ORIENTED_EDGE('',*,*,#3354,.F.);
#4570=ORIENTED_EDGE('',*,*,#3356,.F.);
#4571=ORIENTED_EDGE('',*,*,#3358,.F.);
#4572=ORIENTED_EDGE('',*,*,#3347,.T.);
#4573=ORIENTED_EDGE('',*,*,#3319,.T.);
#4574=ORIENTED_EDGE('',*,*,#3332,.T.);
#4575=ORIENTED_EDGE('',*,*,#3327,.T.);
#4576=ORIENTED_EDGE('',*,*,#3323,.T.);
#4577=ORIENTED_EDGE('',*,*,#3359,.T.);
#4578=ORIENTED_EDGE('',*,*,#3360,.T.);
#4579=ORIENTED_EDGE('',*,*,#3361,.F.);
#4580=ORIENTED_EDGE('',*,*,#3362,.T.);
#4581=ORIENTED_EDGE('',*,*,#3363,.F.);
#4582=ORIENTED_EDGE('',*,*,#3364,.T.);
#4583=ORIENTED_EDGE('',*,*,#3365,.F.);
#4584=ORIENTED_EDGE('',*,*,#3366,.T.);
#4585=ORIENTED_EDGE('',*,*,#3367,.F.);
#4586=ORIENTED_EDGE('',*,*,#3368,.T.);
#4587=ORIENTED_EDGE('',*,*,#3369,.F.);
#4588=ORIENTED_EDGE('',*,*,#3370,.T.);
#4589=ORIENTED_EDGE('',*,*,#3371,.F.);
#4590=ORIENTED_EDGE('',*,*,#3372,.T.);
#4591=ORIENTED_EDGE('',*,*,#3373,.F.);
#4592=ORIENTED_EDGE('',*,*,#3374,.T.);
#4593=ORIENTED_EDGE('',*,*,#3375,.F.);
#4594=ORIENTED_EDGE('',*,*,#3376,.T.);
#4595=ORIENTED_EDGE('',*,*,#3377,.F.);
#4596=ORIENTED_EDGE('',*,*,#3378,.T.);
#4597=ORIENTED_EDGE('',*,*,#3379,.F.);
#4598=ORIENTED_EDGE('',*,*,#3380,.T.);
#4599=ORIENTED_EDGE('',*,*,#3381,.F.);
#4600=ORIENTED_EDGE('',*,*,#3382,.T.);
#4601=ORIENTED_EDGE('',*,*,#3383,.F.);
#4602=ORIENTED_EDGE('',*,*,#3384,.T.);
#4603=ORIENTED_EDGE('',*,*,#3385,.F.);
#4604=ORIENTED_EDGE('',*,*,#3386,.T.);
#4605=ORIENTED_EDGE('',*,*,#3387,.F.);
#4606=ORIENTED_EDGE('',*,*,#3388,.T.);
#4607=ORIENTED_EDGE('',*,*,#3389,.F.);
#4608=ORIENTED_EDGE('',*,*,#3390,.T.);
#4609=ORIENTED_EDGE('',*,*,#3391,.F.);
#4610=ORIENTED_EDGE('',*,*,#3392,.T.);
#4611=ORIENTED_EDGE('',*,*,#3393,.F.);
#4612=ORIENTED_EDGE('',*,*,#3394,.T.);
#4613=ORIENTED_EDGE('',*,*,#3395,.F.);
#4614=ORIENTED_EDGE('',*,*,#3396,.T.);
#4615=ORIENTED_EDGE('',*,*,#3397,.F.);
#4616=ORIENTED_EDGE('',*,*,#3398,.T.);
#4617=ORIENTED_EDGE('',*,*,#3399,.F.);
#4618=ORIENTED_EDGE('',*,*,#3400,.T.);
#4619=ORIENTED_EDGE('',*,*,#3401,.F.);
#4620=ORIENTED_EDGE('',*,*,#3402,.T.);
#4621=ORIENTED_EDGE('',*,*,#3403,.F.);
#4622=ORIENTED_EDGE('',*,*,#3404,.T.);
#4623=ORIENTED_EDGE('',*,*,#3405,.F.);
#4624=ORIENTED_EDGE('',*,*,#3406,.T.);
#4625=ORIENTED_EDGE('',*,*,#3407,.F.);
#4626=ORIENTED_EDGE('',*,*,#3408,.T.);
#4627=ORIENTED_EDGE('',*,*,#3409,.F.);
#4628=ORIENTED_EDGE('',*,*,#3410,.T.);
#4629=ORIENTED_EDGE('',*,*,#3411,.F.);
#4630=ORIENTED_EDGE('',*,*,#3412,.T.);
#4631=ORIENTED_EDGE('',*,*,#3413,.F.);
#4632=ORIENTED_EDGE('',*,*,#3414,.T.);
#4633=ORIENTED_EDGE('',*,*,#3415,.F.);
#4634=ORIENTED_EDGE('',*,*,#3416,.T.);
#4635=ORIENTED_EDGE('',*,*,#3417,.F.);
#4636=ORIENTED_EDGE('',*,*,#3418,.T.);
#4637=ORIENTED_EDGE('',*,*,#3419,.F.);
#4638=ORIENTED_EDGE('',*,*,#3420,.T.);
#4639=ORIENTED_EDGE('',*,*,#3421,.F.);
#4640=ORIENTED_EDGE('',*,*,#3422,.T.);
#4641=ORIENTED_EDGE('',*,*,#3423,.F.);
#4642=ORIENTED_EDGE('',*,*,#3424,.T.);
#4643=ORIENTED_EDGE('',*,*,#3425,.F.);
#4644=ORIENTED_EDGE('',*,*,#3426,.T.);
#4645=ORIENTED_EDGE('',*,*,#3427,.F.);
#4646=ORIENTED_EDGE('',*,*,#3428,.T.);
#4647=ORIENTED_EDGE('',*,*,#3429,.F.);
#4648=ORIENTED_EDGE('',*,*,#3430,.T.);
#4649=ORIENTED_EDGE('',*,*,#3431,.F.);
#4650=ORIENTED_EDGE('',*,*,#3432,.T.);
#4651=ORIENTED_EDGE('',*,*,#3433,.F.);
#4652=ORIENTED_EDGE('',*,*,#3434,.T.);
#4653=ORIENTED_EDGE('',*,*,#3435,.F.);
#4654=ORIENTED_EDGE('',*,*,#3436,.T.);
#4655=ORIENTED_EDGE('',*,*,#3437,.F.);
#4656=ORIENTED_EDGE('',*,*,#3438,.T.);
#4657=ORIENTED_EDGE('',*,*,#3439,.F.);
#4658=ORIENTED_EDGE('',*,*,#3440,.F.);
#4659=ORIENTED_EDGE('',*,*,#3441,.T.);
#4660=ORIENTED_EDGE('',*,*,#3359,.F.);
#4661=ORIENTED_EDGE('',*,*,#3441,.F.);
#4662=ORIENTED_EDGE('',*,*,#3440,.T.);
#4663=ORIENTED_EDGE('',*,*,#3350,.T.);
#4664=ORIENTED_EDGE('',*,*,#3442,.F.);
#4665=ORIENTED_EDGE('',*,*,#3443,.T.);
#4666=ORIENTED_EDGE('',*,*,#3444,.T.);
#4667=ORIENTED_EDGE('',*,*,#3445,.T.);
#4668=ORIENTED_EDGE('',*,*,#3446,.T.);
#4669=ORIENTED_EDGE('',*,*,#3447,.T.);
#4670=ORIENTED_EDGE('',*,*,#3448,.T.);
#4671=ORIENTED_EDGE('',*,*,#3449,.T.);
#4672=ORIENTED_EDGE('',*,*,#3450,.T.);
#4673=ORIENTED_EDGE('',*,*,#3451,.T.);
#4674=ORIENTED_EDGE('',*,*,#3452,.T.);
#4675=ORIENTED_EDGE('',*,*,#3453,.T.);
#4676=ORIENTED_EDGE('',*,*,#3454,.T.);
#4677=ORIENTED_EDGE('',*,*,#3455,.T.);
#4678=ORIENTED_EDGE('',*,*,#3456,.T.);
#4679=ORIENTED_EDGE('',*,*,#3457,.T.);
#4680=ORIENTED_EDGE('',*,*,#3458,.T.);
#4681=ORIENTED_EDGE('',*,*,#3459,.T.);
#4682=ORIENTED_EDGE('',*,*,#3460,.T.);
#4683=ORIENTED_EDGE('',*,*,#3461,.T.);
#4684=ORIENTED_EDGE('',*,*,#3462,.T.);
#4685=ORIENTED_EDGE('',*,*,#3463,.T.);
#4686=ORIENTED_EDGE('',*,*,#3464,.T.);
#4687=ORIENTED_EDGE('',*,*,#3465,.T.);
#4688=ORIENTED_EDGE('',*,*,#3466,.T.);
#4689=ORIENTED_EDGE('',*,*,#3467,.T.);
#4690=ORIENTED_EDGE('',*,*,#3468,.T.);
#4691=ORIENTED_EDGE('',*,*,#3469,.T.);
#4692=ORIENTED_EDGE('',*,*,#3470,.T.);
#4693=ORIENTED_EDGE('',*,*,#3471,.T.);
#4694=ORIENTED_EDGE('',*,*,#3472,.T.);
#4695=ORIENTED_EDGE('',*,*,#3473,.T.);
#4696=ORIENTED_EDGE('',*,*,#3474,.T.);
#4697=ORIENTED_EDGE('',*,*,#3475,.T.);
#4698=ORIENTED_EDGE('',*,*,#3476,.T.);
#4699=ORIENTED_EDGE('',*,*,#3477,.T.);
#4700=ORIENTED_EDGE('',*,*,#3478,.T.);
#4701=ORIENTED_EDGE('',*,*,#3479,.T.);
#4702=ORIENTED_EDGE('',*,*,#3480,.T.);
#4703=ORIENTED_EDGE('',*,*,#3481,.T.);
#4704=ORIENTED_EDGE('',*,*,#3482,.T.);
#4705=ORIENTED_EDGE('',*,*,#3483,.T.);
#4706=ORIENTED_EDGE('',*,*,#3484,.T.);
#4707=ORIENTED_EDGE('',*,*,#3485,.T.);
#4708=ORIENTED_EDGE('',*,*,#3486,.T.);
#4709=ORIENTED_EDGE('',*,*,#3487,.T.);
#4710=ORIENTED_EDGE('',*,*,#3488,.T.);
#4711=ORIENTED_EDGE('',*,*,#3489,.T.);
#4712=ORIENTED_EDGE('',*,*,#3490,.T.);
#4713=ORIENTED_EDGE('',*,*,#3491,.T.);
#4714=ORIENTED_EDGE('',*,*,#3492,.T.);
#4715=ORIENTED_EDGE('',*,*,#3493,.T.);
#4716=ORIENTED_EDGE('',*,*,#3494,.T.);
#4717=ORIENTED_EDGE('',*,*,#3495,.T.);
#4718=ORIENTED_EDGE('',*,*,#3496,.T.);
#4719=ORIENTED_EDGE('',*,*,#3497,.T.);
#4720=ORIENTED_EDGE('',*,*,#3498,.T.);
#4721=ORIENTED_EDGE('',*,*,#3499,.T.);
#4722=ORIENTED_EDGE('',*,*,#3500,.T.);
#4723=ORIENTED_EDGE('',*,*,#3501,.T.);
#4724=ORIENTED_EDGE('',*,*,#3502,.T.);
#4725=ORIENTED_EDGE('',*,*,#3503,.T.);
#4726=ORIENTED_EDGE('',*,*,#3504,.T.);
#4727=ORIENTED_EDGE('',*,*,#3505,.T.);
#4728=ORIENTED_EDGE('',*,*,#3506,.T.);
#4729=ORIENTED_EDGE('',*,*,#3507,.T.);
#4730=ORIENTED_EDGE('',*,*,#3508,.T.);
#4731=ORIENTED_EDGE('',*,*,#3509,.T.);
#4732=ORIENTED_EDGE('',*,*,#3510,.T.);
#4733=ORIENTED_EDGE('',*,*,#3511,.T.);
#4734=ORIENTED_EDGE('',*,*,#3512,.T.);
#4735=ORIENTED_EDGE('',*,*,#3513,.T.);
#4736=ORIENTED_EDGE('',*,*,#3514,.T.);
#4737=ORIENTED_EDGE('',*,*,#3515,.T.);
#4738=ORIENTED_EDGE('',*,*,#3516,.T.);
#4739=ORIENTED_EDGE('',*,*,#3517,.T.);
#4740=ORIENTED_EDGE('',*,*,#3518,.T.);
#4741=ORIENTED_EDGE('',*,*,#3519,.T.);
#4742=ORIENTED_EDGE('',*,*,#3520,.T.);
#4743=ORIENTED_EDGE('',*,*,#3521,.T.);
#4744=ORIENTED_EDGE('',*,*,#3522,.T.);
#4745=ORIENTED_EDGE('',*,*,#3330,.F.);
#4746=ORIENTED_EDGE('',*,*,#3523,.T.);
#4747=ORIENTED_EDGE('',*,*,#3442,.T.);
#4748=ORIENTED_EDGE('',*,*,#3523,.F.);
#4749=ORIENTED_EDGE('',*,*,#3524,.F.);
#4750=ORIENTED_EDGE('',*,*,#3443,.F.);
#4751=ORIENTED_EDGE('',*,*,#3525,.F.);
#4752=ORIENTED_EDGE('',*,*,#3360,.F.);
#4753=ORIENTED_EDGE('',*,*,#3525,.T.);
#4754=ORIENTED_EDGE('',*,*,#3522,.F.);
#4755=ORIENTED_EDGE('',*,*,#3526,.T.);
#4756=ORIENTED_EDGE('',*,*,#3361,.T.);
#4757=ORIENTED_EDGE('',*,*,#3526,.F.);
#4758=ORIENTED_EDGE('',*,*,#3521,.F.);
#4759=ORIENTED_EDGE('',*,*,#3527,.F.);
#4760=ORIENTED_EDGE('',*,*,#3362,.F.);
#4761=ORIENTED_EDGE('',*,*,#3527,.T.);
#4762=ORIENTED_EDGE('',*,*,#3520,.F.);
#4763=ORIENTED_EDGE('',*,*,#3528,.T.);
#4764=ORIENTED_EDGE('',*,*,#3363,.T.);
#4765=ORIENTED_EDGE('',*,*,#3528,.F.);
#4766=ORIENTED_EDGE('',*,*,#3519,.F.);
#4767=ORIENTED_EDGE('',*,*,#3529,.F.);
#4768=ORIENTED_EDGE('',*,*,#3364,.F.);
#4769=ORIENTED_EDGE('',*,*,#3529,.T.);
#4770=ORIENTED_EDGE('',*,*,#3518,.F.);
#4771=ORIENTED_EDGE('',*,*,#3530,.T.);
#4772=ORIENTED_EDGE('',*,*,#3365,.T.);
#4773=ORIENTED_EDGE('',*,*,#3530,.F.);
#4774=ORIENTED_EDGE('',*,*,#3517,.F.);
#4775=ORIENTED_EDGE('',*,*,#3531,.F.);
#4776=ORIENTED_EDGE('',*,*,#3366,.F.);
#4777=ORIENTED_EDGE('',*,*,#3531,.T.);
#4778=ORIENTED_EDGE('',*,*,#3516,.F.);
#4779=ORIENTED_EDGE('',*,*,#3532,.T.);
#4780=ORIENTED_EDGE('',*,*,#3367,.T.);
#4781=ORIENTED_EDGE('',*,*,#3532,.F.);
#4782=ORIENTED_EDGE('',*,*,#3515,.F.);
#4783=ORIENTED_EDGE('',*,*,#3533,.F.);
#4784=ORIENTED_EDGE('',*,*,#3368,.F.);
#4785=ORIENTED_EDGE('',*,*,#3533,.T.);
#4786=ORIENTED_EDGE('',*,*,#3514,.F.);
#4787=ORIENTED_EDGE('',*,*,#3534,.T.);
#4788=ORIENTED_EDGE('',*,*,#3369,.T.);
#4789=ORIENTED_EDGE('',*,*,#3534,.F.);
#4790=ORIENTED_EDGE('',*,*,#3513,.F.);
#4791=ORIENTED_EDGE('',*,*,#3535,.F.);
#4792=ORIENTED_EDGE('',*,*,#3370,.F.);
#4793=ORIENTED_EDGE('',*,*,#3535,.T.);
#4794=ORIENTED_EDGE('',*,*,#3512,.F.);
#4795=ORIENTED_EDGE('',*,*,#3536,.T.);
#4796=ORIENTED_EDGE('',*,*,#3371,.T.);
#4797=ORIENTED_EDGE('',*,*,#3536,.F.);
#4798=ORIENTED_EDGE('',*,*,#3511,.F.);
#4799=ORIENTED_EDGE('',*,*,#3537,.F.);
#4800=ORIENTED_EDGE('',*,*,#3372,.F.);
#4801=ORIENTED_EDGE('',*,*,#3537,.T.);
#4802=ORIENTED_EDGE('',*,*,#3510,.F.);
#4803=ORIENTED_EDGE('',*,*,#3538,.T.);
#4804=ORIENTED_EDGE('',*,*,#3373,.T.);
#4805=ORIENTED_EDGE('',*,*,#3538,.F.);
#4806=ORIENTED_EDGE('',*,*,#3509,.F.);
#4807=ORIENTED_EDGE('',*,*,#3539,.F.);
#4808=ORIENTED_EDGE('',*,*,#3374,.F.);
#4809=ORIENTED_EDGE('',*,*,#3539,.T.);
#4810=ORIENTED_EDGE('',*,*,#3508,.F.);
#4811=ORIENTED_EDGE('',*,*,#3540,.T.);
#4812=ORIENTED_EDGE('',*,*,#3375,.T.);
#4813=ORIENTED_EDGE('',*,*,#3540,.F.);
#4814=ORIENTED_EDGE('',*,*,#3507,.F.);
#4815=ORIENTED_EDGE('',*,*,#3541,.F.);
#4816=ORIENTED_EDGE('',*,*,#3376,.F.);
#4817=ORIENTED_EDGE('',*,*,#3541,.T.);
#4818=ORIENTED_EDGE('',*,*,#3506,.F.);
#4819=ORIENTED_EDGE('',*,*,#3542,.T.);
#4820=ORIENTED_EDGE('',*,*,#3377,.T.);
#4821=ORIENTED_EDGE('',*,*,#3542,.F.);
#4822=ORIENTED_EDGE('',*,*,#3505,.F.);
#4823=ORIENTED_EDGE('',*,*,#3543,.F.);
#4824=ORIENTED_EDGE('',*,*,#3378,.F.);
#4825=ORIENTED_EDGE('',*,*,#3543,.T.);
#4826=ORIENTED_EDGE('',*,*,#3504,.F.);
#4827=ORIENTED_EDGE('',*,*,#3544,.T.);
#4828=ORIENTED_EDGE('',*,*,#3379,.T.);
#4829=ORIENTED_EDGE('',*,*,#3544,.F.);
#4830=ORIENTED_EDGE('',*,*,#3503,.F.);
#4831=ORIENTED_EDGE('',*,*,#3545,.F.);
#4832=ORIENTED_EDGE('',*,*,#3380,.F.);
#4833=ORIENTED_EDGE('',*,*,#3545,.T.);
#4834=ORIENTED_EDGE('',*,*,#3502,.F.);
#4835=ORIENTED_EDGE('',*,*,#3546,.T.);
#4836=ORIENTED_EDGE('',*,*,#3381,.T.);
#4837=ORIENTED_EDGE('',*,*,#3546,.F.);
#4838=ORIENTED_EDGE('',*,*,#3501,.F.);
#4839=ORIENTED_EDGE('',*,*,#3547,.F.);
#4840=ORIENTED_EDGE('',*,*,#3382,.F.);
#4841=ORIENTED_EDGE('',*,*,#3547,.T.);
#4842=ORIENTED_EDGE('',*,*,#3500,.F.);
#4843=ORIENTED_EDGE('',*,*,#3548,.T.);
#4844=ORIENTED_EDGE('',*,*,#3383,.T.);
#4845=ORIENTED_EDGE('',*,*,#3548,.F.);
#4846=ORIENTED_EDGE('',*,*,#3499,.F.);
#4847=ORIENTED_EDGE('',*,*,#3549,.F.);
#4848=ORIENTED_EDGE('',*,*,#3384,.F.);
#4849=ORIENTED_EDGE('',*,*,#3549,.T.);
#4850=ORIENTED_EDGE('',*,*,#3498,.F.);
#4851=ORIENTED_EDGE('',*,*,#3550,.T.);
#4852=ORIENTED_EDGE('',*,*,#3385,.T.);
#4853=ORIENTED_EDGE('',*,*,#3550,.F.);
#4854=ORIENTED_EDGE('',*,*,#3497,.F.);
#4855=ORIENTED_EDGE('',*,*,#3551,.F.);
#4856=ORIENTED_EDGE('',*,*,#3386,.F.);
#4857=ORIENTED_EDGE('',*,*,#3551,.T.);
#4858=ORIENTED_EDGE('',*,*,#3496,.F.);
#4859=ORIENTED_EDGE('',*,*,#3552,.T.);
#4860=ORIENTED_EDGE('',*,*,#3387,.T.);
#4861=ORIENTED_EDGE('',*,*,#3552,.F.);
#4862=ORIENTED_EDGE('',*,*,#3495,.F.);
#4863=ORIENTED_EDGE('',*,*,#3553,.F.);
#4864=ORIENTED_EDGE('',*,*,#3388,.F.);
#4865=ORIENTED_EDGE('',*,*,#3553,.T.);
#4866=ORIENTED_EDGE('',*,*,#3494,.F.);
#4867=ORIENTED_EDGE('',*,*,#3554,.T.);
#4868=ORIENTED_EDGE('',*,*,#3389,.T.);
#4869=ORIENTED_EDGE('',*,*,#3554,.F.);
#4870=ORIENTED_EDGE('',*,*,#3493,.F.);
#4871=ORIENTED_EDGE('',*,*,#3555,.F.);
#4872=ORIENTED_EDGE('',*,*,#3390,.F.);
#4873=ORIENTED_EDGE('',*,*,#3555,.T.);
#4874=ORIENTED_EDGE('',*,*,#3492,.F.);
#4875=ORIENTED_EDGE('',*,*,#3556,.T.);
#4876=ORIENTED_EDGE('',*,*,#3391,.T.);
#4877=ORIENTED_EDGE('',*,*,#3556,.F.);
#4878=ORIENTED_EDGE('',*,*,#3491,.F.);
#4879=ORIENTED_EDGE('',*,*,#3557,.F.);
#4880=ORIENTED_EDGE('',*,*,#3392,.F.);
#4881=ORIENTED_EDGE('',*,*,#3557,.T.);
#4882=ORIENTED_EDGE('',*,*,#3490,.F.);
#4883=ORIENTED_EDGE('',*,*,#3558,.T.);
#4884=ORIENTED_EDGE('',*,*,#3393,.T.);
#4885=ORIENTED_EDGE('',*,*,#3558,.F.);
#4886=ORIENTED_EDGE('',*,*,#3489,.F.);
#4887=ORIENTED_EDGE('',*,*,#3559,.F.);
#4888=ORIENTED_EDGE('',*,*,#3394,.F.);
#4889=ORIENTED_EDGE('',*,*,#3559,.T.);
#4890=ORIENTED_EDGE('',*,*,#3488,.F.);
#4891=ORIENTED_EDGE('',*,*,#3560,.T.);
#4892=ORIENTED_EDGE('',*,*,#3395,.T.);
#4893=ORIENTED_EDGE('',*,*,#3560,.F.);
#4894=ORIENTED_EDGE('',*,*,#3487,.F.);
#4895=ORIENTED_EDGE('',*,*,#3561,.F.);
#4896=ORIENTED_EDGE('',*,*,#3396,.F.);
#4897=ORIENTED_EDGE('',*,*,#3561,.T.);
#4898=ORIENTED_EDGE('',*,*,#3486,.F.);
#4899=ORIENTED_EDGE('',*,*,#3562,.T.);
#4900=ORIENTED_EDGE('',*,*,#3397,.T.);
#4901=ORIENTED_EDGE('',*,*,#3562,.F.);
#4902=ORIENTED_EDGE('',*,*,#3485,.F.);
#4903=ORIENTED_EDGE('',*,*,#3563,.F.);
#4904=ORIENTED_EDGE('',*,*,#3398,.F.);
#4905=ORIENTED_EDGE('',*,*,#3563,.T.);
#4906=ORIENTED_EDGE('',*,*,#3484,.F.);
#4907=ORIENTED_EDGE('',*,*,#3564,.T.);
#4908=ORIENTED_EDGE('',*,*,#3399,.T.);
#4909=ORIENTED_EDGE('',*,*,#3564,.F.);
#4910=ORIENTED_EDGE('',*,*,#3483,.F.);
#4911=ORIENTED_EDGE('',*,*,#3565,.F.);
#4912=ORIENTED_EDGE('',*,*,#3400,.F.);
#4913=ORIENTED_EDGE('',*,*,#3565,.T.);
#4914=ORIENTED_EDGE('',*,*,#3482,.F.);
#4915=ORIENTED_EDGE('',*,*,#3566,.T.);
#4916=ORIENTED_EDGE('',*,*,#3401,.T.);
#4917=ORIENTED_EDGE('',*,*,#3566,.F.);
#4918=ORIENTED_EDGE('',*,*,#3481,.F.);
#4919=ORIENTED_EDGE('',*,*,#3567,.F.);
#4920=ORIENTED_EDGE('',*,*,#3402,.F.);
#4921=ORIENTED_EDGE('',*,*,#3567,.T.);
#4922=ORIENTED_EDGE('',*,*,#3480,.F.);
#4923=ORIENTED_EDGE('',*,*,#3568,.T.);
#4924=ORIENTED_EDGE('',*,*,#3403,.T.);
#4925=ORIENTED_EDGE('',*,*,#3568,.F.);
#4926=ORIENTED_EDGE('',*,*,#3479,.F.);
#4927=ORIENTED_EDGE('',*,*,#3569,.F.);
#4928=ORIENTED_EDGE('',*,*,#3404,.F.);
#4929=ORIENTED_EDGE('',*,*,#3569,.T.);
#4930=ORIENTED_EDGE('',*,*,#3478,.F.);
#4931=ORIENTED_EDGE('',*,*,#3570,.T.);
#4932=ORIENTED_EDGE('',*,*,#3405,.T.);
#4933=ORIENTED_EDGE('',*,*,#3570,.F.);
#4934=ORIENTED_EDGE('',*,*,#3477,.F.);
#4935=ORIENTED_EDGE('',*,*,#3571,.F.);
#4936=ORIENTED_EDGE('',*,*,#3406,.F.);
#4937=ORIENTED_EDGE('',*,*,#3571,.T.);
#4938=ORIENTED_EDGE('',*,*,#3476,.F.);
#4939=ORIENTED_EDGE('',*,*,#3572,.T.);
#4940=ORIENTED_EDGE('',*,*,#3407,.T.);
#4941=ORIENTED_EDGE('',*,*,#3572,.F.);
#4942=ORIENTED_EDGE('',*,*,#3475,.F.);
#4943=ORIENTED_EDGE('',*,*,#3573,.F.);
#4944=ORIENTED_EDGE('',*,*,#3408,.F.);
#4945=ORIENTED_EDGE('',*,*,#3573,.T.);
#4946=ORIENTED_EDGE('',*,*,#3474,.F.);
#4947=ORIENTED_EDGE('',*,*,#3574,.T.);
#4948=ORIENTED_EDGE('',*,*,#3409,.T.);
#4949=ORIENTED_EDGE('',*,*,#3574,.F.);
#4950=ORIENTED_EDGE('',*,*,#3473,.F.);
#4951=ORIENTED_EDGE('',*,*,#3575,.F.);
#4952=ORIENTED_EDGE('',*,*,#3410,.F.);
#4953=ORIENTED_EDGE('',*,*,#3575,.T.);
#4954=ORIENTED_EDGE('',*,*,#3472,.F.);
#4955=ORIENTED_EDGE('',*,*,#3576,.T.);
#4956=ORIENTED_EDGE('',*,*,#3411,.T.);
#4957=ORIENTED_EDGE('',*,*,#3576,.F.);
#4958=ORIENTED_EDGE('',*,*,#3471,.F.);
#4959=ORIENTED_EDGE('',*,*,#3577,.F.);
#4960=ORIENTED_EDGE('',*,*,#3412,.F.);
#4961=ORIENTED_EDGE('',*,*,#3577,.T.);
#4962=ORIENTED_EDGE('',*,*,#3470,.F.);
#4963=ORIENTED_EDGE('',*,*,#3578,.T.);
#4964=ORIENTED_EDGE('',*,*,#3413,.T.);
#4965=ORIENTED_EDGE('',*,*,#3578,.F.);
#4966=ORIENTED_EDGE('',*,*,#3469,.F.);
#4967=ORIENTED_EDGE('',*,*,#3579,.F.);
#4968=ORIENTED_EDGE('',*,*,#3414,.F.);
#4969=ORIENTED_EDGE('',*,*,#3579,.T.);
#4970=ORIENTED_EDGE('',*,*,#3468,.F.);
#4971=ORIENTED_EDGE('',*,*,#3580,.T.);
#4972=ORIENTED_EDGE('',*,*,#3415,.T.);
#4973=ORIENTED_EDGE('',*,*,#3580,.F.);
#4974=ORIENTED_EDGE('',*,*,#3467,.F.);
#4975=ORIENTED_EDGE('',*,*,#3581,.F.);
#4976=ORIENTED_EDGE('',*,*,#3416,.F.);
#4977=ORIENTED_EDGE('',*,*,#3581,.T.);
#4978=ORIENTED_EDGE('',*,*,#3466,.F.);
#4979=ORIENTED_EDGE('',*,*,#3582,.T.);
#4980=ORIENTED_EDGE('',*,*,#3417,.T.);
#4981=ORIENTED_EDGE('',*,*,#3582,.F.);
#4982=ORIENTED_EDGE('',*,*,#3465,.F.);
#4983=ORIENTED_EDGE('',*,*,#3583,.F.);
#4984=ORIENTED_EDGE('',*,*,#3418,.F.);
#4985=ORIENTED_EDGE('',*,*,#3583,.T.);
#4986=ORIENTED_EDGE('',*,*,#3464,.F.);
#4987=ORIENTED_EDGE('',*,*,#3584,.T.);
#4988=ORIENTED_EDGE('',*,*,#3419,.T.);
#4989=ORIENTED_EDGE('',*,*,#3584,.F.);
#4990=ORIENTED_EDGE('',*,*,#3463,.F.);
#4991=ORIENTED_EDGE('',*,*,#3585,.F.);
#4992=ORIENTED_EDGE('',*,*,#3420,.F.);
#4993=ORIENTED_EDGE('',*,*,#3585,.T.);
#4994=ORIENTED_EDGE('',*,*,#3462,.F.);
#4995=ORIENTED_EDGE('',*,*,#3586,.T.);
#4996=ORIENTED_EDGE('',*,*,#3421,.T.);
#4997=ORIENTED_EDGE('',*,*,#3586,.F.);
#4998=ORIENTED_EDGE('',*,*,#3461,.F.);
#4999=ORIENTED_EDGE('',*,*,#3587,.F.);
#5000=ORIENTED_EDGE('',*,*,#3422,.F.);
#5001=ORIENTED_EDGE('',*,*,#3587,.T.);
#5002=ORIENTED_EDGE('',*,*,#3460,.F.);
#5003=ORIENTED_EDGE('',*,*,#3588,.T.);
#5004=ORIENTED_EDGE('',*,*,#3423,.T.);
#5005=ORIENTED_EDGE('',*,*,#3588,.F.);
#5006=ORIENTED_EDGE('',*,*,#3459,.F.);
#5007=ORIENTED_EDGE('',*,*,#3589,.F.);
#5008=ORIENTED_EDGE('',*,*,#3424,.F.);
#5009=ORIENTED_EDGE('',*,*,#3589,.T.);
#5010=ORIENTED_EDGE('',*,*,#3458,.F.);
#5011=ORIENTED_EDGE('',*,*,#3590,.T.);
#5012=ORIENTED_EDGE('',*,*,#3425,.T.);
#5013=ORIENTED_EDGE('',*,*,#3590,.F.);
#5014=ORIENTED_EDGE('',*,*,#3457,.F.);
#5015=ORIENTED_EDGE('',*,*,#3591,.F.);
#5016=ORIENTED_EDGE('',*,*,#3426,.F.);
#5017=ORIENTED_EDGE('',*,*,#3591,.T.);
#5018=ORIENTED_EDGE('',*,*,#3456,.F.);
#5019=ORIENTED_EDGE('',*,*,#3592,.T.);
#5020=ORIENTED_EDGE('',*,*,#3427,.T.);
#5021=ORIENTED_EDGE('',*,*,#3592,.F.);
#5022=ORIENTED_EDGE('',*,*,#3455,.F.);
#5023=ORIENTED_EDGE('',*,*,#3593,.F.);
#5024=ORIENTED_EDGE('',*,*,#3428,.F.);
#5025=ORIENTED_EDGE('',*,*,#3593,.T.);
#5026=ORIENTED_EDGE('',*,*,#3454,.F.);
#5027=ORIENTED_EDGE('',*,*,#3594,.T.);
#5028=ORIENTED_EDGE('',*,*,#3429,.T.);
#5029=ORIENTED_EDGE('',*,*,#3594,.F.);
#5030=ORIENTED_EDGE('',*,*,#3453,.F.);
#5031=ORIENTED_EDGE('',*,*,#3595,.F.);
#5032=ORIENTED_EDGE('',*,*,#3430,.F.);
#5033=ORIENTED_EDGE('',*,*,#3595,.T.);
#5034=ORIENTED_EDGE('',*,*,#3452,.F.);
#5035=ORIENTED_EDGE('',*,*,#3596,.T.);
#5036=ORIENTED_EDGE('',*,*,#3431,.T.);
#5037=ORIENTED_EDGE('',*,*,#3596,.F.);
#5038=ORIENTED_EDGE('',*,*,#3451,.F.);
#5039=ORIENTED_EDGE('',*,*,#3597,.F.);
#5040=ORIENTED_EDGE('',*,*,#3432,.F.);
#5041=ORIENTED_EDGE('',*,*,#3597,.T.);
#5042=ORIENTED_EDGE('',*,*,#3450,.F.);
#5043=ORIENTED_EDGE('',*,*,#3598,.T.);
#5044=ORIENTED_EDGE('',*,*,#3433,.T.);
#5045=ORIENTED_EDGE('',*,*,#3598,.F.);
#5046=ORIENTED_EDGE('',*,*,#3449,.F.);
#5047=ORIENTED_EDGE('',*,*,#3599,.F.);
#5048=ORIENTED_EDGE('',*,*,#3434,.F.);
#5049=ORIENTED_EDGE('',*,*,#3599,.T.);
#5050=ORIENTED_EDGE('',*,*,#3448,.F.);
#5051=ORIENTED_EDGE('',*,*,#3600,.T.);
#5052=ORIENTED_EDGE('',*,*,#3435,.T.);
#5053=ORIENTED_EDGE('',*,*,#3601,.F.);
#5054=ORIENTED_EDGE('',*,*,#3436,.F.);
#5055=ORIENTED_EDGE('',*,*,#3600,.F.);
#5056=ORIENTED_EDGE('',*,*,#3447,.F.);
#5057=ORIENTED_EDGE('',*,*,#3524,.T.);
#5058=ORIENTED_EDGE('',*,*,#3439,.T.);
#5059=ORIENTED_EDGE('',*,*,#3602,.T.);
#5060=ORIENTED_EDGE('',*,*,#3444,.F.);
#5061=ORIENTED_EDGE('',*,*,#3603,.F.);
#5062=ORIENTED_EDGE('',*,*,#3445,.F.);
#5063=ORIENTED_EDGE('',*,*,#3602,.F.);
#5064=ORIENTED_EDGE('',*,*,#3438,.F.);
#5065=ORIENTED_EDGE('',*,*,#3601,.T.);
#5066=ORIENTED_EDGE('',*,*,#3446,.F.);
#5067=ORIENTED_EDGE('',*,*,#3603,.T.);
#5068=ORIENTED_EDGE('',*,*,#3437,.T.);
#5232=CYLINDRICAL_SURFACE('',#6392,0.6);
#5233=CYLINDRICAL_SURFACE('',#6394,0.125);
#5234=CYLINDRICAL_SURFACE('',#6395,0.125);
#5235=CYLINDRICAL_SURFACE('',#6396,1.);
#5236=CYLINDRICAL_SURFACE('',#6399,0.125);
#5237=CYLINDRICAL_SURFACE('',#6400,0.125);
#5238=CYLINDRICAL_SURFACE('',#6484,1.4);
#5239=CYLINDRICAL_SURFACE('',#6569,1.4);
#5240=CYLINDRICAL_SURFACE('',#6570,0.0555000000000001);
#5241=CYLINDRICAL_SURFACE('',#6571,1.24783954473516);
#5242=CYLINDRICAL_SURFACE('',#6572,0.0555000000000001);
#5243=CYLINDRICAL_SURFACE('',#6573,1.24783954473516);
#5244=CYLINDRICAL_SURFACE('',#6574,0.0555000000000001);
#5245=CYLINDRICAL_SURFACE('',#6575,1.24783954473516);
#5246=CYLINDRICAL_SURFACE('',#6576,0.0555000000000001);
#5247=CYLINDRICAL_SURFACE('',#6577,1.24783954473516);
#5248=CYLINDRICAL_SURFACE('',#6578,0.0555000000000001);
#5249=CYLINDRICAL_SURFACE('',#6579,1.24783954473516);
#5250=CYLINDRICAL_SURFACE('',#6580,0.0555000000000001);
#5251=CYLINDRICAL_SURFACE('',#6581,1.24783954473516);
#5252=CYLINDRICAL_SURFACE('',#6582,0.0555000000000001);
#5253=CYLINDRICAL_SURFACE('',#6583,1.24783954473516);
#5254=CYLINDRICAL_SURFACE('',#6584,0.0555000000000001);
#5255=CYLINDRICAL_SURFACE('',#6585,1.24783954473516);
#5256=CYLINDRICAL_SURFACE('',#6586,0.0555000000000001);
#5257=CYLINDRICAL_SURFACE('',#6587,1.24783954473516);
#5258=CYLINDRICAL_SURFACE('',#6588,0.0555000000000001);
#5259=CYLINDRICAL_SURFACE('',#6589,1.24783954473516);
#5260=CYLINDRICAL_SURFACE('',#6590,0.0555000000000001);
#5261=CYLINDRICAL_SURFACE('',#6591,1.24783954473516);
#5262=CYLINDRICAL_SURFACE('',#6592,0.0555000000000001);
#5263=CYLINDRICAL_SURFACE('',#6593,1.24783954473516);
#5264=CYLINDRICAL_SURFACE('',#6594,0.0555000000000001);
#5265=CYLINDRICAL_SURFACE('',#6595,1.24783954473516);
#5266=CYLINDRICAL_SURFACE('',#6596,0.0555000000000001);
#5267=CYLINDRICAL_SURFACE('',#6597,1.24783954473516);
#5268=CYLINDRICAL_SURFACE('',#6598,0.0555000000000001);
#5269=CYLINDRICAL_SURFACE('',#6599,1.24783954473516);
#5270=CYLINDRICAL_SURFACE('',#6600,0.0555000000000001);
#5271=CYLINDRICAL_SURFACE('',#6601,1.24783954473516);
#5272=CYLINDRICAL_SURFACE('',#6602,0.0555000000000001);
#5273=CYLINDRICAL_SURFACE('',#6603,1.24783954473516);
#5274=CYLINDRICAL_SURFACE('',#6604,0.0555000000000001);
#5275=CYLINDRICAL_SURFACE('',#6605,1.24783954473516);
#5276=CYLINDRICAL_SURFACE('',#6606,0.0555000000000001);
#5277=CYLINDRICAL_SURFACE('',#6607,1.24783954473516);
#5278=CYLINDRICAL_SURFACE('',#6608,0.0555000000000001);
#5279=CYLINDRICAL_SURFACE('',#6609,1.24783954473516);
#5280=CYLINDRICAL_SURFACE('',#6610,0.0555000000000001);
#5281=CYLINDRICAL_SURFACE('',#6611,1.24783954473516);
#5282=CYLINDRICAL_SURFACE('',#6612,0.0555000000000001);
#5283=CYLINDRICAL_SURFACE('',#6613,1.24783954473516);
#5284=CYLINDRICAL_SURFACE('',#6614,0.0555000000000001);
#5285=CYLINDRICAL_SURFACE('',#6615,1.24783954473516);
#5286=CYLINDRICAL_SURFACE('',#6616,0.0555000000000001);
#5287=CYLINDRICAL_SURFACE('',#6617,1.24783954473516);
#5288=CYLINDRICAL_SURFACE('',#6618,0.0555000000000001);
#5289=CYLINDRICAL_SURFACE('',#6619,1.24783954473516);
#5290=CYLINDRICAL_SURFACE('',#6620,0.0555000000000001);
#5291=CYLINDRICAL_SURFACE('',#6621,1.24783954473516);
#5292=CYLINDRICAL_SURFACE('',#6622,0.0555000000000001);
#5293=CYLINDRICAL_SURFACE('',#6623,1.24783954473516);
#5294=CYLINDRICAL_SURFACE('',#6624,0.0555000000000001);
#5295=CYLINDRICAL_SURFACE('',#6625,1.24783954473516);
#5296=CYLINDRICAL_SURFACE('',#6626,0.0555000000000001);
#5297=CYLINDRICAL_SURFACE('',#6627,1.24783954473516);
#5298=CYLINDRICAL_SURFACE('',#6628,0.0555000000000001);
#5299=CYLINDRICAL_SURFACE('',#6629,1.24783954473516);
#5300=CYLINDRICAL_SURFACE('',#6630,0.0555000000000001);
#5301=CYLINDRICAL_SURFACE('',#6631,1.24783954473516);
#5302=CYLINDRICAL_SURFACE('',#6632,0.0555000000000001);
#5303=CYLINDRICAL_SURFACE('',#6633,1.24783954473516);
#5304=CYLINDRICAL_SURFACE('',#6634,0.0555000000000001);
#5305=CYLINDRICAL_SURFACE('',#6635,1.24783954473516);
#5306=CYLINDRICAL_SURFACE('',#6636,0.0555000000000001);
#5307=CYLINDRICAL_SURFACE('',#6637,1.24783954473516);
#5308=CYLINDRICAL_SURFACE('',#6638,0.0555000000000001);
#5309=CYLINDRICAL_SURFACE('',#6639,1.24783954473516);
#5310=CYLINDRICAL_SURFACE('',#6640,0.0555000000000001);
#5311=CYLINDRICAL_SURFACE('',#6641,1.24783954473516);
#5312=CYLINDRICAL_SURFACE('',#6642,0.0555000000000001);
#5313=CYLINDRICAL_SURFACE('',#6643,1.24783954473516);
#5314=CYLINDRICAL_SURFACE('',#6644,0.0555000000000001);
#5315=CYLINDRICAL_SURFACE('',#6645,1.24783954473516);
#5316=CYLINDRICAL_SURFACE('',#6646,0.0555000000000001);
#5317=CYLINDRICAL_SURFACE('',#6647,1.24783954473516);
#5318=CYLINDRICAL_SURFACE('',#6648,0.0555000000000001);
#5319=CYLINDRICAL_SURFACE('',#6649,1.24783954473516);
#5532=ADVANCED_FACE('',(#788),#550,.F.);
#5533=ADVANCED_FACE('',(#789,#421),#551,.F.);
#5534=ADVANCED_FACE('',(#790),#552,.F.);
#5535=ADVANCED_FACE('',(#791,#422),#553,.T.);
#5536=ADVANCED_FACE('',(#792,#423,#424,#425),#5232,.F.);
#5537=ADVANCED_FACE('',(#793),#5233,.F.);
#5538=ADVANCED_FACE('',(#794),#5234,.F.);
#5539=ADVANCED_FACE('',(#795,#426,#427,#428),#5235,.T.);
#5540=ADVANCED_FACE('',(#796),#5236,.F.);
#5541=ADVANCED_FACE('',(#797),#5237,.F.);
#5542=ADVANCED_FACE('',(#798,#429),#554,.F.);
#5543=ADVANCED_FACE('',(#799,#430),#555,.T.);
#5544=ADVANCED_FACE('',(#800),#5238,.T.);
#5545=ADVANCED_FACE('',(#801,#431),#556,.F.);
#5546=ADVANCED_FACE('',(#802,#432),#557,.F.);
#5547=ADVANCED_FACE('',(#803),#5239,.T.);
#5548=ADVANCED_FACE('',(#804),#5240,.F.);
#5549=ADVANCED_FACE('',(#805),#5241,.T.);
#5550=ADVANCED_FACE('',(#806),#5242,.F.);
#5551=ADVANCED_FACE('',(#807),#5243,.T.);
#5552=ADVANCED_FACE('',(#808),#5244,.F.);
#5553=ADVANCED_FACE('',(#809),#5245,.T.);
#5554=ADVANCED_FACE('',(#810),#5246,.F.);
#5555=ADVANCED_FACE('',(#811),#5247,.T.);
#5556=ADVANCED_FACE('',(#812),#5248,.F.);
#5557=ADVANCED_FACE('',(#813),#5249,.T.);
#5558=ADVANCED_FACE('',(#814),#5250,.F.);
#5559=ADVANCED_FACE('',(#815),#5251,.T.);
#5560=ADVANCED_FACE('',(#816),#5252,.F.);
#5561=ADVANCED_FACE('',(#817),#5253,.T.);
#5562=ADVANCED_FACE('',(#818),#5254,.F.);
#5563=ADVANCED_FACE('',(#819),#5255,.T.);
#5564=ADVANCED_FACE('',(#820),#5256,.F.);
#5565=ADVANCED_FACE('',(#821),#5257,.T.);
#5566=ADVANCED_FACE('',(#822),#5258,.F.);
#5567=ADVANCED_FACE('',(#823),#5259,.T.);
#5568=ADVANCED_FACE('',(#824),#5260,.F.);
#5569=ADVANCED_FACE('',(#825),#5261,.T.);
#5570=ADVANCED_FACE('',(#826),#5262,.F.);
#5571=ADVANCED_FACE('',(#827),#5263,.T.);
#5572=ADVANCED_FACE('',(#828),#5264,.F.);
#5573=ADVANCED_FACE('',(#829),#5265,.T.);
#5574=ADVANCED_FACE('',(#830),#5266,.F.);
#5575=ADVANCED_FACE('',(#831),#5267,.T.);
#5576=ADVANCED_FACE('',(#832),#5268,.F.);
#5577=ADVANCED_FACE('',(#833),#5269,.T.);
#5578=ADVANCED_FACE('',(#834),#5270,.F.);
#5579=ADVANCED_FACE('',(#835),#5271,.T.);
#5580=ADVANCED_FACE('',(#836),#5272,.F.);
#5581=ADVANCED_FACE('',(#837),#5273,.T.);
#5582=ADVANCED_FACE('',(#838),#5274,.F.);
#5583=ADVANCED_FACE('',(#839),#5275,.T.);
#5584=ADVANCED_FACE('',(#840),#5276,.F.);
#5585=ADVANCED_FACE('',(#841),#5277,.T.);
#5586=ADVANCED_FACE('',(#842),#5278,.F.);
#5587=ADVANCED_FACE('',(#843),#5279,.T.);
#5588=ADVANCED_FACE('',(#844),#5280,.F.);
#5589=ADVANCED_FACE('',(#845),#5281,.T.);
#5590=ADVANCED_FACE('',(#846),#5282,.F.);
#5591=ADVANCED_FACE('',(#847),#5283,.T.);
#5592=ADVANCED_FACE('',(#848),#5284,.F.);
#5593=ADVANCED_FACE('',(#849),#5285,.T.);
#5594=ADVANCED_FACE('',(#850),#5286,.F.);
#5595=ADVANCED_FACE('',(#851),#5287,.T.);
#5596=ADVANCED_FACE('',(#852),#5288,.F.);
#5597=ADVANCED_FACE('',(#853),#5289,.T.);
#5598=ADVANCED_FACE('',(#854),#5290,.F.);
#5599=ADVANCED_FACE('',(#855),#5291,.T.);
#5600=ADVANCED_FACE('',(#856),#5292,.F.);
#5601=ADVANCED_FACE('',(#857),#5293,.T.);
#5602=ADVANCED_FACE('',(#858),#5294,.F.);
#5603=ADVANCED_FACE('',(#859),#5295,.T.);
#5604=ADVANCED_FACE('',(#860),#5296,.F.);
#5605=ADVANCED_FACE('',(#861),#5297,.T.);
#5606=ADVANCED_FACE('',(#862),#5298,.F.);
#5607=ADVANCED_FACE('',(#863),#5299,.T.);
#5608=ADVANCED_FACE('',(#864),#5300,.F.);
#5609=ADVANCED_FACE('',(#865),#5301,.T.);
#5610=ADVANCED_FACE('',(#866),#5302,.F.);
#5611=ADVANCED_FACE('',(#867),#5303,.T.);
#5612=ADVANCED_FACE('',(#868),#5304,.F.);
#5613=ADVANCED_FACE('',(#869),#5305,.T.);
#5614=ADVANCED_FACE('',(#870),#5306,.F.);
#5615=ADVANCED_FACE('',(#871),#5307,.T.);
#5616=ADVANCED_FACE('',(#872),#5308,.F.);
#5617=ADVANCED_FACE('',(#873),#5309,.T.);
#5618=ADVANCED_FACE('',(#874),#5310,.F.);
#5619=ADVANCED_FACE('',(#875),#5311,.T.);
#5620=ADVANCED_FACE('',(#876),#5312,.F.);
#5621=ADVANCED_FACE('',(#877),#5313,.T.);
#5622=ADVANCED_FACE('',(#878),#5314,.F.);
#5623=ADVANCED_FACE('',(#879),#5315,.T.);
#5624=ADVANCED_FACE('',(#880),#5316,.F.);
#5625=ADVANCED_FACE('',(#881),#5317,.T.);
#5626=ADVANCED_FACE('',(#882),#5318,.F.);
#5627=ADVANCED_FACE('',(#883),#5319,.T.);
#5679=CLOSED_SHELL('',(#5532,#5533,#5534,#5535,#5536,#5537,#5538,#5539,
#5540,#5541,#5542,#5543,#5544,#5545,#5546,#5547,#5548,#5549,#5550,#5551,
#5552,#5553,#5554,#5555,#5556,#5557,#5558,#5559,#5560,#5561,#5562,#5563,
#5564,#5565,#5566,#5567,#5568,#5569,#5570,#5571,#5572,#5573,#5574,#5575,
#5576,#5577,#5578,#5579,#5580,#5581,#5582,#5583,#5584,#5585,#5586,#5587,
#5588,#5589,#5590,#5591,#5592,#5593,#5594,#5595,#5596,#5597,#5598,#5599,
#5600,#5601,#5602,#5603,#5604,#5605,#5606,#5607,#5608,#5609,#5610,#5611,
#5612,#5613,#5614,#5615,#5616,#5617,#5618,#5619,#5620,#5621,#5622,#5623,
#5624,#5625,#5626,#5627));
#6384=AXIS2_PLACEMENT_3D('',#9978,#7805,#7806);
#6385=AXIS2_PLACEMENT_3D('',#9979,#7807,#7808);
#6386=AXIS2_PLACEMENT_3D('',#9988,#7813,#7814);
#6387=AXIS2_PLACEMENT_3D('',#9995,#7818,#7819);
#6388=AXIS2_PLACEMENT_3D('',#9996,#7820,#7821);
#6389=AXIS2_PLACEMENT_3D('',#10002,#7825,#7826);
#6390=AXIS2_PLACEMENT_3D('',#10004,#7827,#7828);
#6391=AXIS2_PLACEMENT_3D('',#10005,#7829,#7830);
#6392=AXIS2_PLACEMENT_3D('',#10006,#7831,#7832);
#6393=AXIS2_PLACEMENT_3D('',#10007,#7833,#7834);
#6394=AXIS2_PLACEMENT_3D('',#10122,#7835,#7836);
#6395=AXIS2_PLACEMENT_3D('',#10165,#7838,#7839);
#6396=AXIS2_PLACEMENT_3D('',#10208,#7841,#7842);
#6397=AXIS2_PLACEMENT_3D('',#10210,#7843,#7844);
#6398=AXIS2_PLACEMENT_3D('',#10214,#7847,#7848);
#6399=AXIS2_PLACEMENT_3D('',#10297,#7849,#7850);
#6400=AXIS2_PLACEMENT_3D('',#10299,#7852,#7853);
#6401=AXIS2_PLACEMENT_3D('',#10301,#7855,#7856);
#6402=AXIS2_PLACEMENT_3D('',#10302,#7857,#7858);
#6403=AXIS2_PLACEMENT_3D('',#10304,#7859,#7860);
#6404=AXIS2_PLACEMENT_3D('',#10307,#7861,#7862);
#6405=AXIS2_PLACEMENT_3D('',#10309,#7863,#7864);
#6406=AXIS2_PLACEMENT_3D('',#10311,#7865,#7866);
#6407=AXIS2_PLACEMENT_3D('',#10313,#7867,#7868);
#6408=AXIS2_PLACEMENT_3D('',#10315,#7869,#7870);
#6409=AXIS2_PLACEMENT_3D('',#10317,#7871,#7872);
#6410=AXIS2_PLACEMENT_3D('',#10319,#7873,#7874);
#6411=AXIS2_PLACEMENT_3D('',#10321,#7875,#7876);
#6412=AXIS2_PLACEMENT_3D('',#10323,#7877,#7878);
#6413=AXIS2_PLACEMENT_3D('',#10325,#7879,#7880);
#6414=AXIS2_PLACEMENT_3D('',#10327,#7881,#7882);
#6415=AXIS2_PLACEMENT_3D('',#10329,#7883,#7884);
#6416=AXIS2_PLACEMENT_3D('',#10331,#7885,#7886);
#6417=AXIS2_PLACEMENT_3D('',#10333,#7887,#7888);
#6418=AXIS2_PLACEMENT_3D('',#10335,#7889,#7890);
#6419=AXIS2_PLACEMENT_3D('',#10337,#7891,#7892);
#6420=AXIS2_PLACEMENT_3D('',#10339,#7893,#7894);
#6421=AXIS2_PLACEMENT_3D('',#10341,#7895,#7896);
#6422=AXIS2_PLACEMENT_3D('',#10343,#7897,#7898);
#6423=AXIS2_PLACEMENT_3D('',#10345,#7899,#7900);
#6424=AXIS2_PLACEMENT_3D('',#10347,#7901,#7902);
#6425=AXIS2_PLACEMENT_3D('',#10349,#7903,#7904);
#6426=AXIS2_PLACEMENT_3D('',#10351,#7905,#7906);
#6427=AXIS2_PLACEMENT_3D('',#10353,#7907,#7908);
#6428=AXIS2_PLACEMENT_3D('',#10355,#7909,#7910);
#6429=AXIS2_PLACEMENT_3D('',#10357,#7911,#7912);
#6430=AXIS2_PLACEMENT_3D('',#10359,#7913,#7914);
#6431=AXIS2_PLACEMENT_3D('',#10361,#7915,#7916);
#6432=AXIS2_PLACEMENT_3D('',#10363,#7917,#7918);
#6433=AXIS2_PLACEMENT_3D('',#10365,#7919,#7920);
#6434=AXIS2_PLACEMENT_3D('',#10367,#7921,#7922);
#6435=AXIS2_PLACEMENT_3D('',#10369,#7923,#7924);
#6436=AXIS2_PLACEMENT_3D('',#10371,#7925,#7926);
#6437=AXIS2_PLACEMENT_3D('',#10373,#7927,#7928);
#6438=AXIS2_PLACEMENT_3D('',#10375,#7929,#7930);
#6439=AXIS2_PLACEMENT_3D('',#10377,#7931,#7932);
#6440=AXIS2_PLACEMENT_3D('',#10379,#7933,#7934);
#6441=AXIS2_PLACEMENT_3D('',#10381,#7935,#7936);
#6442=AXIS2_PLACEMENT_3D('',#10383,#7937,#7938);
#6443=AXIS2_PLACEMENT_3D('',#10385,#7939,#7940);
#6444=AXIS2_PLACEMENT_3D('',#10387,#7941,#7942);
#6445=AXIS2_PLACEMENT_3D('',#10389,#7943,#7944);
#6446=AXIS2_PLACEMENT_3D('',#10391,#7945,#7946);
#6447=AXIS2_PLACEMENT_3D('',#10393,#7947,#7948);
#6448=AXIS2_PLACEMENT_3D('',#10395,#7949,#7950);
#6449=AXIS2_PLACEMENT_3D('',#10397,#7951,#7952);
#6450=AXIS2_PLACEMENT_3D('',#10399,#7953,#7954);
#6451=AXIS2_PLACEMENT_3D('',#10401,#7955,#7956);
#6452=AXIS2_PLACEMENT_3D('',#10403,#7957,#7958);
#6453=AXIS2_PLACEMENT_3D('',#10405,#7959,#7960);
#6454=AXIS2_PLACEMENT_3D('',#10407,#7961,#7962);
#6455=AXIS2_PLACEMENT_3D('',#10409,#7963,#7964);
#6456=AXIS2_PLACEMENT_3D('',#10411,#7965,#7966);
#6457=AXIS2_PLACEMENT_3D('',#10413,#7967,#7968);
#6458=AXIS2_PLACEMENT_3D('',#10415,#7969,#7970);
#6459=AXIS2_PLACEMENT_3D('',#10417,#7971,#7972);
#6460=AXIS2_PLACEMENT_3D('',#10419,#7973,#7974);
#6461=AXIS2_PLACEMENT_3D('',#10421,#7975,#7976);
#6462=AXIS2_PLACEMENT_3D('',#10423,#7977,#7978);
#6463=AXIS2_PLACEMENT_3D('',#10425,#7979,#7980);
#6464=AXIS2_PLACEMENT_3D('',#10427,#7981,#7982);
#6465=AXIS2_PLACEMENT_3D('',#10429,#7983,#7984);
#6466=AXIS2_PLACEMENT_3D('',#10431,#7985,#7986);
#6467=AXIS2_PLACEMENT_3D('',#10433,#7987,#7988);
#6468=AXIS2_PLACEMENT_3D('',#10435,#7989,#7990);
#6469=AXIS2_PLACEMENT_3D('',#10437,#7991,#7992);
#6470=AXIS2_PLACEMENT_3D('',#10439,#7993,#7994);
#6471=AXIS2_PLACEMENT_3D('',#10441,#7995,#7996);
#6472=AXIS2_PLACEMENT_3D('',#10443,#7997,#7998);
#6473=AXIS2_PLACEMENT_3D('',#10445,#7999,#8000);
#6474=AXIS2_PLACEMENT_3D('',#10447,#8001,#8002);
#6475=AXIS2_PLACEMENT_3D('',#10449,#8003,#8004);
#6476=AXIS2_PLACEMENT_3D('',#10451,#8005,#8006);
#6477=AXIS2_PLACEMENT_3D('',#10453,#8007,#8008);
#6478=AXIS2_PLACEMENT_3D('',#10455,#8009,#8010);
#6479=AXIS2_PLACEMENT_3D('',#10457,#8011,#8012);
#6480=AXIS2_PLACEMENT_3D('',#10459,#8013,#8014);
#6481=AXIS2_PLACEMENT_3D('',#10461,#8015,#8016);
#6482=AXIS2_PLACEMENT_3D('',#10463,#8017,#8018);
#6483=AXIS2_PLACEMENT_3D('',#10464,#8019,#8020);
#6484=AXIS2_PLACEMENT_3D('',#10465,#8021,#8022);
#6485=AXIS2_PLACEMENT_3D('',#10467,#8023,#8024);
#6486=AXIS2_PLACEMENT_3D('',#10469,#8026,#8027);
#6487=AXIS2_PLACEMENT_3D('',#10470,#8028,#8029);
#6488=AXIS2_PLACEMENT_3D('',#10472,#8030,#8031);
#6489=AXIS2_PLACEMENT_3D('',#10475,#8032,#8033);
#6490=AXIS2_PLACEMENT_3D('',#10477,#8034,#8035);
#6491=AXIS2_PLACEMENT_3D('',#10479,#8036,#8037);
#6492=AXIS2_PLACEMENT_3D('',#10481,#8038,#8039);
#6493=AXIS2_PLACEMENT_3D('',#10483,#8040,#8041);
#6494=AXIS2_PLACEMENT_3D('',#10485,#8042,#8043);
#6495=AXIS2_PLACEMENT_3D('',#10487,#8044,#8045);
#6496=AXIS2_PLACEMENT_3D('',#10489,#8046,#8047);
#6497=AXIS2_PLACEMENT_3D('',#10491,#8048,#8049);
#6498=AXIS2_PLACEMENT_3D('',#10493,#8050,#8051);
#6499=AXIS2_PLACEMENT_3D('',#10495,#8052,#8053);
#6500=AXIS2_PLACEMENT_3D('',#10497,#8054,#8055);
#6501=AXIS2_PLACEMENT_3D('',#10499,#8056,#8057);
#6502=AXIS2_PLACEMENT_3D('',#10501,#8058,#8059);
#6503=AXIS2_PLACEMENT_3D('',#10503,#8060,#8061);
#6504=AXIS2_PLACEMENT_3D('',#10505,#8062,#8063);
#6505=AXIS2_PLACEMENT_3D('',#10507,#8064,#8065);
#6506=AXIS2_PLACEMENT_3D('',#10509,#8066,#8067);
#6507=AXIS2_PLACEMENT_3D('',#10511,#8068,#8069);
#6508=AXIS2_PLACEMENT_3D('',#10513,#8070,#8071);
#6509=AXIS2_PLACEMENT_3D('',#10515,#8072,#8073);
#6510=AXIS2_PLACEMENT_3D('',#10517,#8074,#8075);
#6511=AXIS2_PLACEMENT_3D('',#10519,#8076,#8077);
#6512=AXIS2_PLACEMENT_3D('',#10521,#8078,#8079);
#6513=AXIS2_PLACEMENT_3D('',#10523,#8080,#8081);
#6514=AXIS2_PLACEMENT_3D('',#10525,#8082,#8083);
#6515=AXIS2_PLACEMENT_3D('',#10527,#8084,#8085);
#6516=AXIS2_PLACEMENT_3D('',#10529,#8086,#8087);
#6517=AXIS2_PLACEMENT_3D('',#10531,#8088,#8089);
#6518=AXIS2_PLACEMENT_3D('',#10533,#8090,#8091);
#6519=AXIS2_PLACEMENT_3D('',#10535,#8092,#8093);
#6520=AXIS2_PLACEMENT_3D('',#10537,#8094,#8095);
#6521=AXIS2_PLACEMENT_3D('',#10539,#8096,#8097);
#6522=AXIS2_PLACEMENT_3D('',#10541,#8098,#8099);
#6523=AXIS2_PLACEMENT_3D('',#10543,#8100,#8101);
#6524=AXIS2_PLACEMENT_3D('',#10545,#8102,#8103);
#6525=AXIS2_PLACEMENT_3D('',#10547,#8104,#8105);
#6526=AXIS2_PLACEMENT_3D('',#10549,#8106,#8107);
#6527=AXIS2_PLACEMENT_3D('',#10551,#8108,#8109);
#6528=AXIS2_PLACEMENT_3D('',#10553,#8110,#8111);
#6529=AXIS2_PLACEMENT_3D('',#10555,#8112,#8113);
#6530=AXIS2_PLACEMENT_3D('',#10557,#8114,#8115);
#6531=AXIS2_PLACEMENT_3D('',#10559,#8116,#8117);
#6532=AXIS2_PLACEMENT_3D('',#10561,#8118,#8119);
#6533=AXIS2_PLACEMENT_3D('',#10563,#8120,#8121);
#6534=AXIS2_PLACEMENT_3D('',#10565,#8122,#8123);
#6535=AXIS2_PLACEMENT_3D('',#10567,#8124,#8125);
#6536=AXIS2_PLACEMENT_3D('',#10569,#8126,#8127);
#6537=AXIS2_PLACEMENT_3D('',#10571,#8128,#8129);
#6538=AXIS2_PLACEMENT_3D('',#10573,#8130,#8131);
#6539=AXIS2_PLACEMENT_3D('',#10575,#8132,#8133);
#6540=AXIS2_PLACEMENT_3D('',#10577,#8134,#8135);
#6541=AXIS2_PLACEMENT_3D('',#10579,#8136,#8137);
#6542=AXIS2_PLACEMENT_3D('',#10581,#8138,#8139);
#6543=AXIS2_PLACEMENT_3D('',#10583,#8140,#8141);
#6544=AXIS2_PLACEMENT_3D('',#10585,#8142,#8143);
#6545=AXIS2_PLACEMENT_3D('',#10587,#8144,#8145);
#6546=AXIS2_PLACEMENT_3D('',#10589,#8146,#8147);
#6547=AXIS2_PLACEMENT_3D('',#10591,#8148,#8149);
#6548=AXIS2_PLACEMENT_3D('',#10593,#8150,#8151);
#6549=AXIS2_PLACEMENT_3D('',#10595,#8152,#8153);
#6550=AXIS2_PLACEMENT_3D('',#10597,#8154,#8155);
#6551=AXIS2_PLACEMENT_3D('',#10599,#8156,#8157);
#6552=AXIS2_PLACEMENT_3D('',#10601,#8158,#8159);
#6553=AXIS2_PLACEMENT_3D('',#10603,#8160,#8161);
#6554=AXIS2_PLACEMENT_3D('',#10605,#8162,#8163);
#6555=AXIS2_PLACEMENT_3D('',#10607,#8164,#8165);
#6556=AXIS2_PLACEMENT_3D('',#10609,#8166,#8167);
#6557=AXIS2_PLACEMENT_3D('',#10611,#8168,#8169);
#6558=AXIS2_PLACEMENT_3D('',#10613,#8170,#8171);
#6559=AXIS2_PLACEMENT_3D('',#10615,#8172,#8173);
#6560=AXIS2_PLACEMENT_3D('',#10617,#8174,#8175);
#6561=AXIS2_PLACEMENT_3D('',#10619,#8176,#8177);
#6562=AXIS2_PLACEMENT_3D('',#10621,#8178,#8179);
#6563=AXIS2_PLACEMENT_3D('',#10623,#8180,#8181);
#6564=AXIS2_PLACEMENT_3D('',#10625,#8182,#8183);
#6565=AXIS2_PLACEMENT_3D('',#10627,#8184,#8185);
#6566=AXIS2_PLACEMENT_3D('',#10629,#8186,#8187);
#6567=AXIS2_PLACEMENT_3D('',#10631,#8188,#8189);
#6568=AXIS2_PLACEMENT_3D('',#10632,#8190,#8191);
#6569=AXIS2_PLACEMENT_3D('',#10633,#8192,#8193);
#6570=AXIS2_PLACEMENT_3D('',#10635,#8195,#8196);
#6571=AXIS2_PLACEMENT_3D('',#10638,#8199,#8200);
#6572=AXIS2_PLACEMENT_3D('',#10640,#8202,#8203);
#6573=AXIS2_PLACEMENT_3D('',#10642,#8205,#8206);
#6574=AXIS2_PLACEMENT_3D('',#10644,#8208,#8209);
#6575=AXIS2_PLACEMENT_3D('',#10646,#8211,#8212);
#6576=AXIS2_PLACEMENT_3D('',#10648,#8214,#8215);
#6577=AXIS2_PLACEMENT_3D('',#10650,#8217,#8218);
#6578=AXIS2_PLACEMENT_3D('',#10652,#8220,#8221);
#6579=AXIS2_PLACEMENT_3D('',#10654,#8223,#8224);
#6580=AXIS2_PLACEMENT_3D('',#10656,#8226,#8227);
#6581=AXIS2_PLACEMENT_3D('',#10658,#8229,#8230);
#6582=AXIS2_PLACEMENT_3D('',#10660,#8232,#8233);
#6583=AXIS2_PLACEMENT_3D('',#10662,#8235,#8236);
#6584=AXIS2_PLACEMENT_3D('',#10664,#8238,#8239);
#6585=AXIS2_PLACEMENT_3D('',#10666,#8241,#8242);
#6586=AXIS2_PLACEMENT_3D('',#10668,#8244,#8245);
#6587=AXIS2_PLACEMENT_3D('',#10670,#8247,#8248);
#6588=AXIS2_PLACEMENT_3D('',#10672,#8250,#8251);
#6589=AXIS2_PLACEMENT_3D('',#10674,#8253,#8254);
#6590=AXIS2_PLACEMENT_3D('',#10676,#8256,#8257);
#6591=AXIS2_PLACEMENT_3D('',#10678,#8259,#8260);
#6592=AXIS2_PLACEMENT_3D('',#10680,#8262,#8263);
#6593=AXIS2_PLACEMENT_3D('',#10682,#8265,#8266);
#6594=AXIS2_PLACEMENT_3D('',#10684,#8268,#8269);
#6595=AXIS2_PLACEMENT_3D('',#10686,#8271,#8272);
#6596=AXIS2_PLACEMENT_3D('',#10688,#8274,#8275);
#6597=AXIS2_PLACEMENT_3D('',#10690,#8277,#8278);
#6598=AXIS2_PLACEMENT_3D('',#10692,#8280,#8281);
#6599=AXIS2_PLACEMENT_3D('',#10694,#8283,#8284);
#6600=AXIS2_PLACEMENT_3D('',#10696,#8286,#8287);
#6601=AXIS2_PLACEMENT_3D('',#10698,#8289,#8290);
#6602=AXIS2_PLACEMENT_3D('',#10700,#8292,#8293);
#6603=AXIS2_PLACEMENT_3D('',#10702,#8295,#8296);
#6604=AXIS2_PLACEMENT_3D('',#10704,#8298,#8299);
#6605=AXIS2_PLACEMENT_3D('',#10706,#8301,#8302);
#6606=AXIS2_PLACEMENT_3D('',#10708,#8304,#8305);
#6607=AXIS2_PLACEMENT_3D('',#10710,#8307,#8308);
#6608=AXIS2_PLACEMENT_3D('',#10712,#8310,#8311);
#6609=AXIS2_PLACEMENT_3D('',#10714,#8313,#8314);
#6610=AXIS2_PLACEMENT_3D('',#10716,#8316,#8317);
#6611=AXIS2_PLACEMENT_3D('',#10718,#8319,#8320);
#6612=AXIS2_PLACEMENT_3D('',#10720,#8322,#8323);
#6613=AXIS2_PLACEMENT_3D('',#10722,#8325,#8326);
#6614=AXIS2_PLACEMENT_3D('',#10724,#8328,#8329);
#6615=AXIS2_PLACEMENT_3D('',#10726,#8331,#8332);
#6616=AXIS2_PLACEMENT_3D('',#10728,#8334,#8335);
#6617=AXIS2_PLACEMENT_3D('',#10730,#8337,#8338);
#6618=AXIS2_PLACEMENT_3D('',#10732,#8340,#8341);
#6619=AXIS2_PLACEMENT_3D('',#10734,#8343,#8344);
#6620=AXIS2_PLACEMENT_3D('',#10736,#8346,#8347);
#6621=AXIS2_PLACEMENT_3D('',#10738,#8349,#8350);
#6622=AXIS2_PLACEMENT_3D('',#10740,#8352,#8353);
#6623=AXIS2_PLACEMENT_3D('',#10742,#8355,#8356);
#6624=AXIS2_PLACEMENT_3D('',#10744,#8358,#8359);
#6625=AXIS2_PLACEMENT_3D('',#10746,#8361,#8362);
#6626=AXIS2_PLACEMENT_3D('',#10748,#8364,#8365);
#6627=AXIS2_PLACEMENT_3D('',#10750,#8367,#8368);
#6628=AXIS2_PLACEMENT_3D('',#10752,#8370,#8371);
#6629=AXIS2_PLACEMENT_3D('',#10754,#8373,#8374);
#6630=AXIS2_PLACEMENT_3D('',#10756,#8376,#8377);
#6631=AXIS2_PLACEMENT_3D('',#10758,#8379,#8380);
#6632=AXIS2_PLACEMENT_3D('',#10760,#8382,#8383);
#6633=AXIS2_PLACEMENT_3D('',#10762,#8385,#8386);
#6634=AXIS2_PLACEMENT_3D('',#10764,#8388,#8389);
#6635=AXIS2_PLACEMENT_3D('',#10766,#8391,#8392);
#6636=AXIS2_PLACEMENT_3D('',#10768,#8394,#8395);
#6637=AXIS2_PLACEMENT_3D('',#10770,#8397,#8398);
#6638=AXIS2_PLACEMENT_3D('',#10772,#8400,#8401);
#6639=AXIS2_PLACEMENT_3D('',#10774,#8403,#8404);
#6640=AXIS2_PLACEMENT_3D('',#10776,#8406,#8407);
#6641=AXIS2_PLACEMENT_3D('',#10778,#8409,#8410);
#6642=AXIS2_PLACEMENT_3D('',#10780,#8412,#8413);
#6643=AXIS2_PLACEMENT_3D('',#10782,#8415,#8416);
#6644=AXIS2_PLACEMENT_3D('',#10784,#8418,#8419);
#6645=AXIS2_PLACEMENT_3D('',#10786,#8421,#8422);
#6646=AXIS2_PLACEMENT_3D('',#10788,#8424,#8425);
#6647=AXIS2_PLACEMENT_3D('',#10790,#8427,#8428);
#6648=AXIS2_PLACEMENT_3D('',#10792,#8430,#8431);
#6649=AXIS2_PLACEMENT_3D('',#10794,#8433,#8434);
#7805=DIRECTION('axis',(0.,0.,1.));
#7806=DIRECTION('refdir',(1.,0.,0.));
#7807=DIRECTION('center_axis',(-1.,0.,0.));
#7808=DIRECTION('ref_axis',(0.,0.,1.));
#7809=DIRECTION('',(0.,0.,1.));
#7810=DIRECTION('',(0.,1.,0.));
#7811=DIRECTION('',(0.,0.,-1.));
#7812=DIRECTION('',(0.,1.,0.));
#7813=DIRECTION('center_axis',(0.,0.,-1.));
#7814=DIRECTION('ref_axis',(-1.,0.,0.));
#7815=DIRECTION('',(-1.,0.,0.));
#7816=DIRECTION('',(0.,1.,0.));
#7817=DIRECTION('',(1.,0.,0.));
#7818=DIRECTION('center_axis',(0.,0.,1.));
#7819=DIRECTION('ref_axis',(1.,0.,0.));
#7820=DIRECTION('center_axis',(1.,0.,0.));
#7821=DIRECTION('ref_axis',(0.,0.,-1.));
#7822=DIRECTION('',(0.,0.,-1.));
#7823=DIRECTION('',(0.,-1.,0.));
#7824=DIRECTION('',(0.,0.,1.));
#7825=DIRECTION('center_axis',(0.,1.,0.));
#7826=DIRECTION('ref_axis',(1.,0.,0.));
#7827=DIRECTION('center_axis',(0.,1.,0.));
#7828=DIRECTION('ref_axis',(1.,0.,0.));
#7829=DIRECTION('center_axis',(0.,-1.,0.));
#7830=DIRECTION('ref_axis',(1.,0.,0.));
#7831=DIRECTION('center_axis',(0.,1.,0.));
#7832=DIRECTION('ref_axis',(-1.83697019872103E-16,0.,1.));
#7833=DIRECTION('center_axis',(0.,1.,0.));
#7834=DIRECTION('ref_axis',(1.,0.,0.));
#7835=DIRECTION('center_axis',(1.,0.,6.12323399573677E-17));
#7836=DIRECTION('ref_axis',(6.12323399573677E-17,0.,-1.));
#7837=DIRECTION('',(1.,0.,6.12323399573677E-17));
#7838=DIRECTION('center_axis',(1.,0.,6.12323399573677E-17));
#7839=DIRECTION('ref_axis',(6.12323399573677E-17,0.,-1.));
#7840=DIRECTION('',(1.,0.,6.12323399573677E-17));
#7841=DIRECTION('center_axis',(0.,-1.,0.));
#7842=DIRECTION('ref_axis',(1.,0.,0.));
#7843=DIRECTION('center_axis',(0.,-1.,0.));
#7844=DIRECTION('ref_axis',(1.,0.,0.));
#7845=DIRECTION('',(0.,1.,0.));
#7846=DIRECTION('',(0.,1.,0.));
#7847=DIRECTION('center_axis',(0.,1.,0.));
#7848=DIRECTION('ref_axis',(1.,0.,0.));
#7849=DIRECTION('center_axis',(0.,0.,1.));
#7850=DIRECTION('ref_axis',(1.,0.,0.));
#7851=DIRECTION('',(0.,0.,1.));
#7852=DIRECTION('center_axis',(0.,0.,1.));
#7853=DIRECTION('ref_axis',(1.,0.,0.));
#7854=DIRECTION('',(0.,0.,1.));
#7855=DIRECTION('center_axis',(0.,1.,0.));
#7856=DIRECTION('ref_axis',(1.,0.,0.));
#7857=DIRECTION('center_axis',(0.,1.,0.));
#7858=DIRECTION('ref_axis',(1.,0.,0.));
#7859=DIRECTION('center_axis',(0.,1.,0.));
#7860=DIRECTION('ref_axis',(1.,0.,0.));
#7861=DIRECTION('center_axis',(0.,1.,0.));
#7862=DIRECTION('ref_axis',(0.987688340595138,0.,0.156434465040231));
#7863=DIRECTION('center_axis',(0.,1.,0.));
#7864=DIRECTION('ref_axis',(1.,0.,0.));
#7865=DIRECTION('center_axis',(0.,1.,0.));
#7866=DIRECTION('ref_axis',(0.951056516295154,0.,0.309016994374948));
#7867=DIRECTION('center_axis',(0.,1.,0.));
#7868=DIRECTION('ref_axis',(1.,0.,0.));
#7869=DIRECTION('center_axis',(0.,1.,0.));
#7870=DIRECTION('ref_axis',(0.891006524188368,0.,0.453990499739547));
#7871=DIRECTION('center_axis',(0.,1.,0.));
#7872=DIRECTION('ref_axis',(1.,0.,0.));
#7873=DIRECTION('center_axis',(0.,1.,0.));
#7874=DIRECTION('ref_axis',(0.809016994374947,0.,0.587785252292473));
#7875=DIRECTION('center_axis',(0.,1.,0.));
#7876=DIRECTION('ref_axis',(1.,0.,0.));
#7877=DIRECTION('center_axis',(0.,1.,0.));
#7878=DIRECTION('ref_axis',(0.707106781186547,0.,0.707106781186548));
#7879=DIRECTION('center_axis',(0.,1.,0.));
#7880=DIRECTION('ref_axis',(1.,0.,0.));
#7881=DIRECTION('center_axis',(0.,1.,0.));
#7882=DIRECTION('ref_axis',(0.587785252292473,0.,0.809016994374948));
#7883=DIRECTION('center_axis',(0.,1.,0.));
#7884=DIRECTION('ref_axis',(1.,0.,0.));
#7885=DIRECTION('center_axis',(0.,1.,0.));
#7886=DIRECTION('ref_axis',(0.453990499739547,0.,0.891006524188368));
#7887=DIRECTION('center_axis',(0.,1.,0.));
#7888=DIRECTION('ref_axis',(1.,0.,0.));
#7889=DIRECTION('center_axis',(0.,1.,0.));
#7890=DIRECTION('ref_axis',(0.309016994374947,0.,0.951056516295154));
#7891=DIRECTION('center_axis',(0.,1.,0.));
#7892=DIRECTION('ref_axis',(1.,0.,0.));
#7893=DIRECTION('center_axis',(0.,1.,0.));
#7894=DIRECTION('ref_axis',(0.156434465040231,0.,0.987688340595138));
#7895=DIRECTION('center_axis',(0.,1.,0.));
#7896=DIRECTION('ref_axis',(1.,0.,0.));
#7897=DIRECTION('center_axis',(0.,1.,0.));
#7898=DIRECTION('ref_axis',(-1.83697019872103E-16,0.,1.));
#7899=DIRECTION('center_axis',(0.,1.,0.));
#7900=DIRECTION('ref_axis',(1.,0.,0.));
#7901=DIRECTION('center_axis',(0.,1.,0.));
#7902=DIRECTION('ref_axis',(-0.156434465040231,0.,0.987688340595138));
#7903=DIRECTION('center_axis',(0.,1.,0.));
#7904=DIRECTION('ref_axis',(1.,0.,0.));
#7905=DIRECTION('center_axis',(0.,1.,0.));
#7906=DIRECTION('ref_axis',(-0.309016994374948,0.,0.951056516295154));
#7907=DIRECTION('center_axis',(0.,1.,0.));
#7908=DIRECTION('ref_axis',(1.,0.,0.));
#7909=DIRECTION('center_axis',(0.,1.,0.));
#7910=DIRECTION('ref_axis',(-0.453990499739547,0.,0.891006524188368));
#7911=DIRECTION('center_axis',(0.,1.,0.));
#7912=DIRECTION('ref_axis',(1.,0.,0.));
#7913=DIRECTION('center_axis',(0.,1.,0.));
#7914=DIRECTION('ref_axis',(-0.587785252292473,0.,0.809016994374947));
#7915=DIRECTION('center_axis',(0.,1.,0.));
#7916=DIRECTION('ref_axis',(1.,0.,0.));
#7917=DIRECTION('center_axis',(0.,1.,0.));
#7918=DIRECTION('ref_axis',(-0.707106781186548,0.,0.707106781186547));
#7919=DIRECTION('center_axis',(0.,1.,0.));
#7920=DIRECTION('ref_axis',(1.,0.,0.));
#7921=DIRECTION('center_axis',(0.,1.,0.));
#7922=DIRECTION('ref_axis',(-0.809016994374947,0.,0.587785252292473));
#7923=DIRECTION('center_axis',(0.,1.,0.));
#7924=DIRECTION('ref_axis',(1.,0.,0.));
#7925=DIRECTION('center_axis',(0.,1.,0.));
#7926=DIRECTION('ref_axis',(-0.891006524188368,0.,0.453990499739547));
#7927=DIRECTION('center_axis',(0.,1.,0.));
#7928=DIRECTION('ref_axis',(1.,0.,0.));
#7929=DIRECTION('center_axis',(0.,1.,0.));
#7930=DIRECTION('ref_axis',(-0.951056516295154,0.,0.309016994374947));
#7931=DIRECTION('center_axis',(0.,1.,0.));
#7932=DIRECTION('ref_axis',(1.,0.,0.));
#7933=DIRECTION('center_axis',(0.,1.,0.));
#7934=DIRECTION('ref_axis',(-0.987688340595138,0.,0.156434465040231));
#7935=DIRECTION('center_axis',(0.,1.,0.));
#7936=DIRECTION('ref_axis',(1.,0.,0.));
#7937=DIRECTION('center_axis',(0.,1.,0.));
#7938=DIRECTION('ref_axis',(-1.,0.,-1.22464679914735E-16));
#7939=DIRECTION('center_axis',(0.,1.,0.));
#7940=DIRECTION('ref_axis',(1.,0.,0.));
#7941=DIRECTION('center_axis',(0.,1.,0.));
#7942=DIRECTION('ref_axis',(-0.987688340595138,0.,-0.156434465040231));
#7943=DIRECTION('center_axis',(0.,1.,0.));
#7944=DIRECTION('ref_axis',(1.,0.,0.));
#7945=DIRECTION('center_axis',(0.,1.,0.));
#7946=DIRECTION('ref_axis',(-0.951056516295154,0.,-0.309016994374948));
#7947=DIRECTION('center_axis',(0.,1.,0.));
#7948=DIRECTION('ref_axis',(1.,0.,0.));
#7949=DIRECTION('center_axis',(0.,1.,0.));
#7950=DIRECTION('ref_axis',(-0.891006524188368,0.,-0.453990499739547));
#7951=DIRECTION('center_axis',(0.,1.,0.));
#7952=DIRECTION('ref_axis',(1.,0.,0.));
#7953=DIRECTION('center_axis',(0.,1.,0.));
#7954=DIRECTION('ref_axis',(-0.809016994374947,0.,-0.587785252292473));
#7955=DIRECTION('center_axis',(0.,1.,0.));
#7956=DIRECTION('ref_axis',(1.,0.,0.));
#7957=DIRECTION('center_axis',(0.,1.,0.));
#7958=DIRECTION('ref_axis',(-0.707106781186547,0.,-0.707106781186548));
#7959=DIRECTION('center_axis',(0.,1.,0.));
#7960=DIRECTION('ref_axis',(1.,0.,0.));
#7961=DIRECTION('center_axis',(0.,1.,0.));
#7962=DIRECTION('ref_axis',(-0.587785252292473,0.,-0.809016994374947));
#7963=DIRECTION('center_axis',(0.,1.,0.));
#7964=DIRECTION('ref_axis',(1.,0.,0.));
#7965=DIRECTION('center_axis',(0.,1.,0.));
#7966=DIRECTION('ref_axis',(-0.453990499739547,0.,-0.891006524188368));
#7967=DIRECTION('center_axis',(0.,1.,0.));
#7968=DIRECTION('ref_axis',(1.,0.,0.));
#7969=DIRECTION('center_axis',(0.,1.,0.));
#7970=DIRECTION('ref_axis',(-0.309016994374947,0.,-0.951056516295154));
#7971=DIRECTION('center_axis',(0.,1.,0.));
#7972=DIRECTION('ref_axis',(1.,0.,0.));
#7973=DIRECTION('center_axis',(0.,1.,0.));
#7974=DIRECTION('ref_axis',(-0.156434465040231,0.,-0.987688340595138));
#7975=DIRECTION('center_axis',(0.,1.,0.));
#7976=DIRECTION('ref_axis',(1.,0.,0.));
#7977=DIRECTION('center_axis',(0.,1.,0.));
#7978=DIRECTION('ref_axis',(6.12323399573677E-17,0.,-1.));
#7979=DIRECTION('center_axis',(0.,1.,0.));
#7980=DIRECTION('ref_axis',(1.,0.,0.));
#7981=DIRECTION('center_axis',(0.,1.,0.));
#7982=DIRECTION('ref_axis',(0.156434465040231,0.,-0.987688340595138));
#7983=DIRECTION('center_axis',(0.,1.,0.));
#7984=DIRECTION('ref_axis',(1.,0.,0.));
#7985=DIRECTION('center_axis',(0.,1.,0.));
#7986=DIRECTION('ref_axis',(0.309016994374948,0.,-0.951056516295154));
#7987=DIRECTION('center_axis',(0.,1.,0.));
#7988=DIRECTION('ref_axis',(1.,0.,0.));
#7989=DIRECTION('center_axis',(0.,1.,0.));
#7990=DIRECTION('ref_axis',(0.453990499739547,0.,-0.891006524188368));
#7991=DIRECTION('center_axis',(0.,1.,0.));
#7992=DIRECTION('ref_axis',(1.,0.,0.));
#7993=DIRECTION('center_axis',(0.,1.,0.));
#7994=DIRECTION('ref_axis',(0.587785252292473,0.,-0.809016994374947));
#7995=DIRECTION('center_axis',(0.,1.,0.));
#7996=DIRECTION('ref_axis',(1.,0.,0.));
#7997=DIRECTION('center_axis',(0.,1.,0.));
#7998=DIRECTION('ref_axis',(0.707106781186548,0.,-0.707106781186547));
#7999=DIRECTION('center_axis',(0.,1.,0.));
#8000=DIRECTION('ref_axis',(1.,0.,0.));
#8001=DIRECTION('center_axis',(0.,1.,0.));
#8002=DIRECTION('ref_axis',(0.809016994374947,0.,-0.587785252292473));
#8003=DIRECTION('center_axis',(0.,1.,0.));
#8004=DIRECTION('ref_axis',(1.,0.,0.));
#8005=DIRECTION('center_axis',(0.,1.,0.));
#8006=DIRECTION('ref_axis',(0.891006524188368,0.,-0.453990499739547));
#8007=DIRECTION('center_axis',(0.,1.,0.));
#8008=DIRECTION('ref_axis',(1.,0.,0.));
#8009=DIRECTION('center_axis',(0.,1.,0.));
#8010=DIRECTION('ref_axis',(0.951056516295154,0.,-0.309016994374947));
#8011=DIRECTION('center_axis',(0.,1.,0.));
#8012=DIRECTION('ref_axis',(1.,0.,0.));
#8013=DIRECTION('center_axis',(0.,1.,0.));
#8014=DIRECTION('ref_axis',(0.987688340595138,0.,-0.156434465040231));
#8015=DIRECTION('center_axis',(0.,1.,0.));
#8016=DIRECTION('ref_axis',(1.,0.,0.));
#8017=DIRECTION('center_axis',(0.,1.,0.));
#8018=DIRECTION('ref_axis',(1.,0.,0.));
#8019=DIRECTION('center_axis',(0.,1.,0.));
#8020=DIRECTION('ref_axis',(1.,0.,0.));
#8021=DIRECTION('center_axis',(0.,-1.,0.));
#8022=DIRECTION('ref_axis',(1.,0.,0.));
#8023=DIRECTION('center_axis',(0.,-1.,0.));
#8024=DIRECTION('ref_axis',(1.,0.,0.));
#8025=DIRECTION('',(0.,1.,0.));
#8026=DIRECTION('center_axis',(0.,1.,0.));
#8027=DIRECTION('ref_axis',(1.,0.,0.));
#8028=DIRECTION('center_axis',(0.,1.,0.));
#8029=DIRECTION('ref_axis',(1.,0.,0.));
#8030=DIRECTION('center_axis',(0.,1.,0.));
#8031=DIRECTION('ref_axis',(1.,0.,0.));
#8032=DIRECTION('center_axis',(0.,-1.,0.));
#8033=DIRECTION('ref_axis',(0.987688340595138,0.,0.156434465040231));
#8034=DIRECTION('center_axis',(0.,1.,0.));
#8035=DIRECTION('ref_axis',(1.,0.,0.));
#8036=DIRECTION('center_axis',(0.,-1.,0.));
#8037=DIRECTION('ref_axis',(1.,0.,0.));
#8038=DIRECTION('center_axis',(0.,1.,0.));
#8039=DIRECTION('ref_axis',(1.,0.,0.));
#8040=DIRECTION('center_axis',(0.,-1.,0.));
#8041=DIRECTION('ref_axis',(0.987688340595138,0.,-0.156434465040231));
#8042=DIRECTION('center_axis',(0.,1.,0.));
#8043=DIRECTION('ref_axis',(1.,0.,0.));
#8044=DIRECTION('center_axis',(0.,-1.,0.));
#8045=DIRECTION('ref_axis',(0.951056516295154,0.,-0.309016994374947));
#8046=DIRECTION('center_axis',(0.,1.,0.));
#8047=DIRECTION('ref_axis',(1.,0.,0.));
#8048=DIRECTION('center_axis',(0.,-1.,0.));
#8049=DIRECTION('ref_axis',(0.891006524188368,0.,-0.453990499739547));
#8050=DIRECTION('center_axis',(0.,1.,0.));
#8051=DIRECTION('ref_axis',(1.,0.,0.));
#8052=DIRECTION('center_axis',(0.,-1.,0.));
#8053=DIRECTION('ref_axis',(0.809016994374947,0.,-0.587785252292473));
#8054=DIRECTION('center_axis',(0.,1.,0.));
#8055=DIRECTION('ref_axis',(1.,0.,0.));
#8056=DIRECTION('center_axis',(0.,-1.,0.));
#8057=DIRECTION('ref_axis',(0.707106781186548,0.,-0.707106781186547));
#8058=DIRECTION('center_axis',(0.,1.,0.));
#8059=DIRECTION('ref_axis',(1.,0.,0.));
#8060=DIRECTION('center_axis',(0.,-1.,0.));
#8061=DIRECTION('ref_axis',(0.587785252292473,0.,-0.809016994374947));
#8062=DIRECTION('center_axis',(0.,1.,0.));
#8063=DIRECTION('ref_axis',(1.,0.,0.));
#8064=DIRECTION('center_axis',(0.,-1.,0.));
#8065=DIRECTION('ref_axis',(0.453990499739547,0.,-0.891006524188368));
#8066=DIRECTION('center_axis',(0.,1.,0.));
#8067=DIRECTION('ref_axis',(1.,0.,0.));
#8068=DIRECTION('center_axis',(0.,-1.,0.));
#8069=DIRECTION('ref_axis',(0.309016994374948,0.,-0.951056516295154));
#8070=DIRECTION('center_axis',(0.,1.,0.));
#8071=DIRECTION('ref_axis',(1.,0.,0.));
#8072=DIRECTION('center_axis',(0.,-1.,0.));
#8073=DIRECTION('ref_axis',(0.156434465040231,0.,-0.987688340595138));
#8074=DIRECTION('center_axis',(0.,1.,0.));
#8075=DIRECTION('ref_axis',(1.,0.,0.));
#8076=DIRECTION('center_axis',(0.,-1.,0.));
#8077=DIRECTION('ref_axis',(6.12323399573677E-17,0.,-1.));
#8078=DIRECTION('center_axis',(0.,1.,0.));
#8079=DIRECTION('ref_axis',(1.,0.,0.));
#8080=DIRECTION('center_axis',(0.,-1.,0.));
#8081=DIRECTION('ref_axis',(-0.156434465040231,0.,-0.987688340595138));
#8082=DIRECTION('center_axis',(0.,1.,0.));
#8083=DIRECTION('ref_axis',(1.,0.,0.));
#8084=DIRECTION('center_axis',(0.,-1.,0.));
#8085=DIRECTION('ref_axis',(-0.309016994374947,0.,-0.951056516295154));
#8086=DIRECTION('center_axis',(0.,1.,0.));
#8087=DIRECTION('ref_axis',(1.,0.,0.));
#8088=DIRECTION('center_axis',(0.,-1.,0.));
#8089=DIRECTION('ref_axis',(-0.453990499739547,0.,-0.891006524188368));
#8090=DIRECTION('center_axis',(0.,1.,0.));
#8091=DIRECTION('ref_axis',(1.,0.,0.));
#8092=DIRECTION('center_axis',(0.,-1.,0.));
#8093=DIRECTION('ref_axis',(-0.587785252292473,0.,-0.809016994374947));
#8094=DIRECTION('center_axis',(0.,1.,0.));
#8095=DIRECTION('ref_axis',(1.,0.,0.));
#8096=DIRECTION('center_axis',(0.,-1.,0.));
#8097=DIRECTION('ref_axis',(-0.707106781186547,0.,-0.707106781186548));
#8098=DIRECTION('center_axis',(0.,1.,0.));
#8099=DIRECTION('ref_axis',(1.,0.,0.));
#8100=DIRECTION('center_axis',(0.,-1.,0.));
#8101=DIRECTION('ref_axis',(-0.809016994374947,0.,-0.587785252292473));
#8102=DIRECTION('center_axis',(0.,1.,0.));
#8103=DIRECTION('ref_axis',(1.,0.,0.));
#8104=DIRECTION('center_axis',(0.,-1.,0.));
#8105=DIRECTION('ref_axis',(-0.891006524188368,0.,-0.453990499739547));
#8106=DIRECTION('center_axis',(0.,1.,0.));
#8107=DIRECTION('ref_axis',(1.,0.,0.));
#8108=DIRECTION('center_axis',(0.,-1.,0.));
#8109=DIRECTION('ref_axis',(-0.951056516295154,0.,-0.309016994374948));
#8110=DIRECTION('center_axis',(0.,1.,0.));
#8111=DIRECTION('ref_axis',(1.,0.,0.));
#8112=DIRECTION('center_axis',(0.,-1.,0.));
#8113=DIRECTION('ref_axis',(-0.987688340595138,0.,-0.156434465040231));
#8114=DIRECTION('center_axis',(0.,1.,0.));
#8115=DIRECTION('ref_axis',(1.,0.,0.));
#8116=DIRECTION('center_axis',(0.,-1.,0.));
#8117=DIRECTION('ref_axis',(-1.,0.,-1.22464679914735E-16));
#8118=DIRECTION('center_axis',(0.,1.,0.));
#8119=DIRECTION('ref_axis',(1.,0.,0.));
#8120=DIRECTION('center_axis',(0.,-1.,0.));
#8121=DIRECTION('ref_axis',(-0.987688340595138,0.,0.156434465040231));
#8122=DIRECTION('center_axis',(0.,1.,0.));
#8123=DIRECTION('ref_axis',(1.,0.,0.));
#8124=DIRECTION('center_axis',(0.,-1.,0.));
#8125=DIRECTION('ref_axis',(-0.951056516295154,0.,0.309016994374947));
#8126=DIRECTION('center_axis',(0.,1.,0.));
#8127=DIRECTION('ref_axis',(1.,0.,0.));
#8128=DIRECTION('center_axis',(0.,-1.,0.));
#8129=DIRECTION('ref_axis',(-0.891006524188368,0.,0.453990499739547));
#8130=DIRECTION('center_axis',(0.,1.,0.));
#8131=DIRECTION('ref_axis',(1.,0.,0.));
#8132=DIRECTION('center_axis',(0.,-1.,0.));
#8133=DIRECTION('ref_axis',(-0.809016994374947,0.,0.587785252292473));
#8134=DIRECTION('center_axis',(0.,1.,0.));
#8135=DIRECTION('ref_axis',(1.,0.,0.));
#8136=DIRECTION('center_axis',(0.,-1.,0.));
#8137=DIRECTION('ref_axis',(-0.707106781186548,0.,0.707106781186547));
#8138=DIRECTION('center_axis',(0.,1.,0.));
#8139=DIRECTION('ref_axis',(1.,0.,0.));
#8140=DIRECTION('center_axis',(0.,-1.,0.));
#8141=DIRECTION('ref_axis',(-0.587785252292473,0.,0.809016994374947));
#8142=DIRECTION('center_axis',(0.,1.,0.));
#8143=DIRECTION('ref_axis',(1.,0.,0.));
#8144=DIRECTION('center_axis',(0.,-1.,0.));
#8145=DIRECTION('ref_axis',(-0.453990499739547,0.,0.891006524188368));
#8146=DIRECTION('center_axis',(0.,1.,0.));
#8147=DIRECTION('ref_axis',(1.,0.,0.));
#8148=DIRECTION('center_axis',(0.,-1.,0.));
#8149=DIRECTION('ref_axis',(-0.309016994374948,0.,0.951056516295154));
#8150=DIRECTION('center_axis',(0.,1.,0.));
#8151=DIRECTION('ref_axis',(1.,0.,0.));
#8152=DIRECTION('center_axis',(0.,-1.,0.));
#8153=DIRECTION('ref_axis',(-0.156434465040231,0.,0.987688340595138));
#8154=DIRECTION('center_axis',(0.,1.,0.));
#8155=DIRECTION('ref_axis',(1.,0.,0.));
#8156=DIRECTION('center_axis',(0.,-1.,0.));
#8157=DIRECTION('ref_axis',(-1.83697019872103E-16,0.,1.));
#8158=DIRECTION('center_axis',(0.,1.,0.));
#8159=DIRECTION('ref_axis',(1.,0.,0.));
#8160=DIRECTION('center_axis',(0.,-1.,0.));
#8161=DIRECTION('ref_axis',(0.156434465040231,0.,0.987688340595138));
#8162=DIRECTION('center_axis',(0.,1.,0.));
#8163=DIRECTION('ref_axis',(1.,0.,0.));
#8164=DIRECTION('center_axis',(0.,-1.,0.));
#8165=DIRECTION('ref_axis',(0.309016994374947,0.,0.951056516295154));
#8166=DIRECTION('center_axis',(0.,1.,0.));
#8167=DIRECTION('ref_axis',(1.,0.,0.));
#8168=DIRECTION('center_axis',(0.,-1.,0.));
#8169=DIRECTION('ref_axis',(0.453990499739547,0.,0.891006524188368));
#8170=DIRECTION('center_axis',(0.,1.,0.));
#8171=DIRECTION('ref_axis',(1.,0.,0.));
#8172=DIRECTION('center_axis',(0.,-1.,0.));
#8173=DIRECTION('ref_axis',(0.587785252292473,0.,0.809016994374948));
#8174=DIRECTION('center_axis',(0.,1.,0.));
#8175=DIRECTION('ref_axis',(1.,0.,0.));
#8176=DIRECTION('center_axis',(0.,-1.,0.));
#8177=DIRECTION('ref_axis',(0.707106781186547,0.,0.707106781186548));
#8178=DIRECTION('center_axis',(0.,1.,0.));
#8179=DIRECTION('ref_axis',(1.,0.,0.));
#8180=DIRECTION('center_axis',(0.,-1.,0.));
#8181=DIRECTION('ref_axis',(0.809016994374947,0.,0.587785252292473));
#8182=DIRECTION('center_axis',(0.,1.,0.));
#8183=DIRECTION('ref_axis',(1.,0.,0.));
#8184=DIRECTION('center_axis',(0.,-1.,0.));
#8185=DIRECTION('ref_axis',(0.891006524188368,0.,0.453990499739547));
#8186=DIRECTION('center_axis',(0.,1.,0.));
#8187=DIRECTION('ref_axis',(1.,0.,0.));
#8188=DIRECTION('center_axis',(0.,-1.,0.));
#8189=DIRECTION('ref_axis',(0.951056516295154,0.,0.309016994374948));
#8190=DIRECTION('center_axis',(0.,1.,0.));
#8191=DIRECTION('ref_axis',(1.,0.,0.));
#8192=DIRECTION('center_axis',(0.,1.,0.));
#8193=DIRECTION('ref_axis',(1.,0.,0.));
#8194=DIRECTION('',(0.,-1.,0.));
#8195=DIRECTION('center_axis',(0.,1.,0.));
#8196=DIRECTION('ref_axis',(-0.987688340595137,0.,-0.156434465040233));
#8197=DIRECTION('',(0.,-1.,0.));
#8198=DIRECTION('',(0.,1.,0.));
#8199=DIRECTION('center_axis',(0.,1.,0.));
#8200=DIRECTION('ref_axis',(1.,0.,0.));
#8201=DIRECTION('',(0.,-1.,0.));
#8202=DIRECTION('center_axis',(0.,1.,0.));
#8203=DIRECTION('ref_axis',(-0.951056516295153,0.,-0.309016994374949));
#8204=DIRECTION('',(0.,1.,0.));
#8205=DIRECTION('center_axis',(0.,1.,0.));
#8206=DIRECTION('ref_axis',(1.,0.,0.));
#8207=DIRECTION('',(0.,-1.,0.));
#8208=DIRECTION('center_axis',(0.,1.,0.));
#8209=DIRECTION('ref_axis',(-0.891006524188368,0.,-0.453990499739547));
#8210=DIRECTION('',(0.,1.,0.));
#8211=DIRECTION('center_axis',(0.,1.,0.));
#8212=DIRECTION('ref_axis',(1.,0.,0.));
#8213=DIRECTION('',(0.,-1.,0.));
#8214=DIRECTION('center_axis',(0.,1.,0.));
#8215=DIRECTION('ref_axis',(-0.809016994374948,0.,-0.587785252292473));
#8216=DIRECTION('',(0.,1.,0.));
#8217=DIRECTION('center_axis',(0.,1.,0.));
#8218=DIRECTION('ref_axis',(1.,0.,0.));
#8219=DIRECTION('',(0.,-1.,0.));
#8220=DIRECTION('center_axis',(0.,1.,0.));
#8221=DIRECTION('ref_axis',(-0.707106781186547,0.,-0.707106781186548));
#8222=DIRECTION('',(0.,1.,0.));
#8223=DIRECTION('center_axis',(0.,1.,0.));
#8224=DIRECTION('ref_axis',(1.,0.,0.));
#8225=DIRECTION('',(0.,-1.,0.));
#8226=DIRECTION('center_axis',(0.,1.,0.));
#8227=DIRECTION('ref_axis',(-0.587785252292474,0.,-0.809016994374947));
#8228=DIRECTION('',(0.,1.,0.));
#8229=DIRECTION('center_axis',(0.,1.,0.));
#8230=DIRECTION('ref_axis',(1.,0.,0.));
#8231=DIRECTION('',(0.,-1.,0.));
#8232=DIRECTION('center_axis',(0.,1.,0.));
#8233=DIRECTION('ref_axis',(-0.453990499739547,0.,-0.891006524188368));
#8234=DIRECTION('',(0.,1.,0.));
#8235=DIRECTION('center_axis',(0.,1.,0.));
#8236=DIRECTION('ref_axis',(1.,0.,0.));
#8237=DIRECTION('',(0.,-1.,0.));
#8238=DIRECTION('center_axis',(0.,1.,0.));
#8239=DIRECTION('ref_axis',(-0.309016994374948,0.,-0.951056516295153));
#8240=DIRECTION('',(0.,1.,0.));
#8241=DIRECTION('center_axis',(0.,1.,0.));
#8242=DIRECTION('ref_axis',(1.,0.,0.));
#8243=DIRECTION('',(0.,-1.,0.));
#8244=DIRECTION('center_axis',(0.,1.,0.));
#8245=DIRECTION('ref_axis',(-0.156434465040232,0.,-0.987688340595138));
#8246=DIRECTION('',(0.,1.,0.));
#8247=DIRECTION('center_axis',(0.,1.,0.));
#8248=DIRECTION('ref_axis',(1.,0.,0.));
#8249=DIRECTION('',(0.,-1.,0.));
#8250=DIRECTION('center_axis',(0.,1.,0.));
#8251=DIRECTION('ref_axis',(3.06161699786838E-16,0.,-1.));
#8252=DIRECTION('',(0.,1.,0.));
#8253=DIRECTION('center_axis',(0.,1.,0.));
#8254=DIRECTION('ref_axis',(1.,0.,0.));
#8255=DIRECTION('',(0.,-1.,0.));
#8256=DIRECTION('center_axis',(0.,1.,0.));
#8257=DIRECTION('ref_axis',(0.156434465040233,0.,-0.987688340595138));
#8258=DIRECTION('',(0.,1.,0.));
#8259=DIRECTION('center_axis',(0.,1.,0.));
#8260=DIRECTION('ref_axis',(1.,0.,0.));
#8261=DIRECTION('',(0.,-1.,0.));
#8262=DIRECTION('center_axis',(0.,1.,0.));
#8263=DIRECTION('ref_axis',(0.309016994374946,0.,-0.951056516295154));
#8264=DIRECTION('',(0.,1.,0.));
#8265=DIRECTION('center_axis',(0.,1.,0.));
#8266=DIRECTION('ref_axis',(1.,0.,0.));
#8267=DIRECTION('',(0.,-1.,0.));
#8268=DIRECTION('center_axis',(0.,1.,0.));
#8269=DIRECTION('ref_axis',(0.453990499739547,0.,-0.891006524188368));
#8270=DIRECTION('',(0.,1.,0.));
#8271=DIRECTION('center_axis',(0.,1.,0.));
#8272=DIRECTION('ref_axis',(1.,0.,0.));
#8273=DIRECTION('',(0.,-1.,0.));
#8274=DIRECTION('center_axis',(0.,1.,0.));
#8275=DIRECTION('ref_axis',(0.587785252292473,0.,-0.809016994374947));
#8276=DIRECTION('',(0.,1.,0.));
#8277=DIRECTION('center_axis',(0.,1.,0.));
#8278=DIRECTION('ref_axis',(1.,0.,0.));
#8279=DIRECTION('',(0.,-1.,0.));
#8280=DIRECTION('center_axis',(0.,1.,0.));
#8281=DIRECTION('ref_axis',(0.707106781186548,0.,-0.707106781186547));
#8282=DIRECTION('',(0.,1.,0.));
#8283=DIRECTION('center_axis',(0.,1.,0.));
#8284=DIRECTION('ref_axis',(1.,0.,0.));
#8285=DIRECTION('',(0.,-1.,0.));
#8286=DIRECTION('center_axis',(0.,1.,0.));
#8287=DIRECTION('ref_axis',(0.809016994374946,0.,-0.587785252292475));
#8288=DIRECTION('',(0.,1.,0.));
#8289=DIRECTION('center_axis',(0.,1.,0.));
#8290=DIRECTION('ref_axis',(1.,0.,0.));
#8291=DIRECTION('',(0.,-1.,0.));
#8292=DIRECTION('center_axis',(0.,1.,0.));
#8293=DIRECTION('ref_axis',(0.891006524188368,0.,-0.453990499739547));
#8294=DIRECTION('',(0.,1.,0.));
#8295=DIRECTION('center_axis',(0.,1.,0.));
#8296=DIRECTION('ref_axis',(1.,0.,0.));
#8297=DIRECTION('',(0.,-1.,0.));
#8298=DIRECTION('center_axis',(0.,1.,0.));
#8299=DIRECTION('ref_axis',(0.951056516295154,0.,-0.309016994374946));
#8300=DIRECTION('',(0.,1.,0.));
#8301=DIRECTION('center_axis',(0.,1.,0.));
#8302=DIRECTION('ref_axis',(1.,0.,0.));
#8303=DIRECTION('',(0.,-1.,0.));
#8304=DIRECTION('center_axis',(0.,1.,0.));
#8305=DIRECTION('ref_axis',(0.987688340595138,0.,-0.156434465040232));
#8306=DIRECTION('',(0.,1.,0.));
#8307=DIRECTION('center_axis',(0.,1.,0.));
#8308=DIRECTION('ref_axis',(1.,0.,0.));
#8309=DIRECTION('',(0.,-1.,0.));
#8310=DIRECTION('center_axis',(0.,1.,0.));
#8311=DIRECTION('ref_axis',(1.,0.,2.44929359829471E-16));
#8312=DIRECTION('',(0.,1.,0.));
#8313=DIRECTION('center_axis',(0.,1.,0.));
#8314=DIRECTION('ref_axis',(1.,0.,0.));
#8315=DIRECTION('',(0.,-1.,0.));
#8316=DIRECTION('center_axis',(0.,1.,0.));
#8317=DIRECTION('ref_axis',(0.987688340595137,0.,0.156434465040232));
#8318=DIRECTION('',(0.,1.,0.));
#8319=DIRECTION('center_axis',(0.,1.,0.));
#8320=DIRECTION('ref_axis',(1.,0.,0.));
#8321=DIRECTION('',(0.,-1.,0.));
#8322=DIRECTION('center_axis',(0.,1.,0.));
#8323=DIRECTION('ref_axis',(0.951056516295154,0.,0.309016994374946));
#8324=DIRECTION('',(0.,1.,0.));
#8325=DIRECTION('center_axis',(0.,1.,0.));
#8326=DIRECTION('ref_axis',(1.,0.,0.));
#8327=DIRECTION('',(0.,-1.,0.));
#8328=DIRECTION('center_axis',(0.,1.,0.));
#8329=DIRECTION('ref_axis',(0.891006524188368,0.,0.453990499739547));
#8330=DIRECTION('',(0.,1.,0.));
#8331=DIRECTION('center_axis',(0.,1.,0.));
#8332=DIRECTION('ref_axis',(1.,0.,0.));
#8333=DIRECTION('',(0.,-1.,0.));
#8334=DIRECTION('center_axis',(0.,1.,0.));
#8335=DIRECTION('ref_axis',(0.809016994374947,0.,0.587785252292473));
#8336=DIRECTION('',(0.,1.,0.));
#8337=DIRECTION('center_axis',(0.,1.,0.));
#8338=DIRECTION('ref_axis',(1.,0.,0.));
#8339=DIRECTION('',(0.,-1.,0.));
#8340=DIRECTION('center_axis',(0.,1.,0.));
#8341=DIRECTION('ref_axis',(0.707106781186547,0.,0.707106781186548));
#8342=DIRECTION('',(0.,1.,0.));
#8343=DIRECTION('center_axis',(0.,1.,0.));
#8344=DIRECTION('ref_axis',(1.,0.,0.));
#8345=DIRECTION('',(0.,-1.,0.));
#8346=DIRECTION('center_axis',(0.,1.,0.));
#8347=DIRECTION('ref_axis',(0.587785252292475,0.,0.809016994374946));
#8348=DIRECTION('',(0.,1.,0.));
#8349=DIRECTION('center_axis',(0.,1.,0.));
#8350=DIRECTION('ref_axis',(1.,0.,0.));
#8351=DIRECTION('',(0.,-1.,0.));
#8352=DIRECTION('center_axis',(0.,1.,0.));
#8353=DIRECTION('ref_axis',(0.453990499739547,0.,0.891006524188368));
#8354=DIRECTION('',(0.,1.,0.));
#8355=DIRECTION('center_axis',(0.,1.,0.));
#8356=DIRECTION('ref_axis',(1.,0.,0.));
#8357=DIRECTION('',(0.,-1.,0.));
#8358=DIRECTION('center_axis',(0.,1.,0.));
#8359=DIRECTION('ref_axis',(0.309016994374946,0.,0.951056516295154));
#8360=DIRECTION('',(0.,1.,0.));
#8361=DIRECTION('center_axis',(0.,1.,0.));
#8362=DIRECTION('ref_axis',(1.,0.,0.));
#8363=DIRECTION('',(0.,-1.,0.));
#8364=DIRECTION('center_axis',(0.,1.,0.));
#8365=DIRECTION('ref_axis',(0.156434465040232,0.,0.987688340595138));
#8366=DIRECTION('',(0.,1.,0.));
#8367=DIRECTION('center_axis',(0.,1.,0.));
#8368=DIRECTION('ref_axis',(1.,0.,0.));
#8369=DIRECTION('',(0.,-1.,0.));
#8370=DIRECTION('center_axis',(0.,1.,0.));
#8371=DIRECTION('ref_axis',(-1.83697019872103E-16,0.,1.));
#8372=DIRECTION('',(0.,1.,0.));
#8373=DIRECTION('center_axis',(0.,1.,0.));
#8374=DIRECTION('ref_axis',(1.,0.,0.));
#8375=DIRECTION('',(0.,-1.,0.));
#8376=DIRECTION('center_axis',(0.,1.,0.));
#8377=DIRECTION('ref_axis',(-0.156434465040232,0.,0.987688340595138));
#8378=DIRECTION('',(0.,1.,0.));
#8379=DIRECTION('center_axis',(0.,1.,0.));
#8380=DIRECTION('ref_axis',(1.,0.,0.));
#8381=DIRECTION('',(0.,-1.,0.));
#8382=DIRECTION('center_axis',(0.,1.,0.));
#8383=DIRECTION('ref_axis',(-0.309016994374946,0.,0.951056516295154));
#8384=DIRECTION('',(0.,1.,0.));
#8385=DIRECTION('center_axis',(0.,1.,0.));
#8386=DIRECTION('ref_axis',(1.,0.,0.));
#8387=DIRECTION('',(0.,-1.,0.));
#8388=DIRECTION('center_axis',(0.,1.,0.));
#8389=DIRECTION('ref_axis',(-0.453990499739549,0.,0.891006524188367));
#8390=DIRECTION('',(0.,1.,0.));
#8391=DIRECTION('center_axis',(0.,1.,0.));
#8392=DIRECTION('ref_axis',(1.,0.,0.));
#8393=DIRECTION('',(0.,-1.,0.));
#8394=DIRECTION('center_axis',(0.,1.,0.));
#8395=DIRECTION('ref_axis',(-0.587785252292474,0.,0.809016994374947));
#8396=DIRECTION('',(0.,1.,0.));
#8397=DIRECTION('center_axis',(0.,1.,0.));
#8398=DIRECTION('ref_axis',(1.,0.,0.));
#8399=DIRECTION('',(0.,-1.,0.));
#8400=DIRECTION('center_axis',(0.,1.,0.));
#8401=DIRECTION('ref_axis',(-0.707106781186548,0.,0.707106781186547));
#8402=DIRECTION('',(0.,1.,0.));
#8403=DIRECTION('center_axis',(0.,1.,0.));
#8404=DIRECTION('ref_axis',(1.,0.,0.));
#8405=DIRECTION('',(0.,-1.,0.));
#8406=DIRECTION('center_axis',(0.,1.,0.));
#8407=DIRECTION('ref_axis',(-0.809016994374947,0.,0.587785252292474));
#8408=DIRECTION('',(0.,1.,0.));
#8409=DIRECTION('center_axis',(0.,1.,0.));
#8410=DIRECTION('ref_axis',(1.,0.,0.));
#8411=DIRECTION('',(0.,-1.,0.));
#8412=DIRECTION('center_axis',(0.,1.,0.));
#8413=DIRECTION('ref_axis',(-0.891006524188368,0.,0.453990499739547));
#8414=DIRECTION('',(0.,1.,0.));
#8415=DIRECTION('center_axis',(0.,1.,0.));
#8416=DIRECTION('ref_axis',(1.,0.,0.));
#8417=DIRECTION('',(0.,-1.,0.));
#8418=DIRECTION('center_axis',(0.,1.,0.));
#8419=DIRECTION('ref_axis',(-0.951056516295154,0.,0.309016994374948));
#8420=DIRECTION('',(0.,1.,0.));
#8421=DIRECTION('center_axis',(0.,1.,0.));
#8422=DIRECTION('ref_axis',(1.,0.,0.));
#8423=DIRECTION('',(0.,-1.,0.));
#8424=DIRECTION('center_axis',(0.,1.,0.));
#8425=DIRECTION('ref_axis',(-0.987688340595137,0.,0.156434465040233));
#8426=DIRECTION('',(0.,1.,0.));
#8427=DIRECTION('center_axis',(0.,1.,0.));
#8428=DIRECTION('ref_axis',(1.,0.,0.));
#8429=DIRECTION('',(0.,1.,0.));
#8430=DIRECTION('center_axis',(0.,1.,0.));
#8431=DIRECTION('ref_axis',(-1.,0.,-1.22464679914735E-16));
#8432=DIRECTION('',(0.,-1.,0.));
#8433=DIRECTION('center_axis',(0.,1.,0.));
#8434=DIRECTION('ref_axis',(1.,0.,0.));
#9978=CARTESIAN_POINT('',(0.,0.,0.));
#9979=CARTESIAN_POINT('Origin',(-0.2,-1.,-0.78));
#9980=CARTESIAN_POINT('',(-0.2,-0.9,-0.78));
#9981=CARTESIAN_POINT('',(-0.2,-0.9,-0.565685424949238));
#9982=CARTESIAN_POINT('',(-0.2,-0.9,-0.39));
#9983=CARTESIAN_POINT('',(-0.2,0.85,-0.78));
#9984=CARTESIAN_POINT('',(-0.2,-1.,-0.78));
#9985=CARTESIAN_POINT('',(-0.2,0.85,-0.565685424949238));
#9986=CARTESIAN_POINT('',(-0.2,0.85,-0.39));
#9987=CARTESIAN_POINT('',(-0.2,0.,-0.565685424949238));
#9988=CARTESIAN_POINT('Origin',(0.2,-1.,-0.78));
#9989=CARTESIAN_POINT('',(0.2,-0.9,-0.78));
#9990=CARTESIAN_POINT('',(0.1,-0.9,-0.78));
#9991=CARTESIAN_POINT('',(0.2,0.85,-0.78));
#9992=CARTESIAN_POINT('',(0.2,-1.,-0.78));
#9993=CARTESIAN_POINT('',(0.1,0.85,-0.78));
#9994=CARTESIAN_POINT('',(-0.125,-0.5,-0.78));
#9995=CARTESIAN_POINT('Origin',(0.,-0.5,-0.78));
#9996=CARTESIAN_POINT('Origin',(0.2,-1.,0.));
#9997=CARTESIAN_POINT('',(0.2,-0.9,-0.565685424949238));
#9998=CARTESIAN_POINT('',(0.2,-0.9,0.));
#9999=CARTESIAN_POINT('',(0.2,0.85,-0.565685424949238));
#10000=CARTESIAN_POINT('',(0.2,0.,-0.565685424949238));
#10001=CARTESIAN_POINT('',(0.2,0.85,0.));
#10002=CARTESIAN_POINT('Origin',(0.,0.85,0.));
#10003=CARTESIAN_POINT('',(-1.4,0.85,1.71450551880629E-16));
#10004=CARTESIAN_POINT('Origin',(0.,0.85,0.));
#10005=CARTESIAN_POINT('Origin',(0.,0.85,0.));
#10006=CARTESIAN_POINT('Origin',(0.,0.,0.));
#10007=CARTESIAN_POINT('Origin',(0.,-0.9,0.));
#10008=CARTESIAN_POINT('',(0.125,-0.5,0.586834729715275));
#10009=CARTESIAN_POINT('',(-0.125,-0.5,0.586834729715275));
#10010=CARTESIAN_POINT('Ctrl Pts',(0.125,-0.5,0.586834729715275));
#10011=CARTESIAN_POINT('Ctrl Pts',(0.125,-0.484254474936005,0.586834729715275));
#10012=CARTESIAN_POINT('Ctrl Pts',(0.121843784097853,-0.467492086231842,
0.587534197873268));
#10013=CARTESIAN_POINT('Ctrl Pts',(0.109073016834181,-0.436709004341607,
0.590038488226116));
#10014=CARTESIAN_POINT('Ctrl Pts',(0.0994608796208941,-0.422684184324257,
0.591804743154611));
#10015=CARTESIAN_POINT('Ctrl Pts',(0.077316548567853,-0.400539853271216,
0.59510289473619));
#10016=CARTESIAN_POINT('Ctrl Pts',(0.0632914182239686,-0.390927142361291,
0.596852269967858));
#10017=CARTESIAN_POINT('Ctrl Pts',(0.0325072544867634,-0.378155958502111,
0.599317707212167));
#10018=CARTESIAN_POINT('Ctrl Pts',(0.0157444828659572,-0.375,0.6));
#10019=CARTESIAN_POINT('Ctrl Pts',(-0.0157444828659573,-0.375,0.6));
#10020=CARTESIAN_POINT('Ctrl Pts',(-0.0325072544867634,-0.378155958502111,
0.599317707212167));
#10021=CARTESIAN_POINT('Ctrl Pts',(-0.0632914182239687,-0.390927142361291,
0.596852269967858));
#10022=CARTESIAN_POINT('Ctrl Pts',(-0.077316548567853,-0.400539853271216,
0.59510289473619));
#10023=CARTESIAN_POINT('Ctrl Pts',(-0.0994608796208942,-0.422684184324257,
0.591804743154611));
#10024=CARTESIAN_POINT('Ctrl Pts',(-0.109073016834181,-0.436709004341607,
0.590038488226116));
#10025=CARTESIAN_POINT('Ctrl Pts',(-0.121843784097853,-0.467492086231842,
0.587534197873268));
#10026=CARTESIAN_POINT('Ctrl Pts',(-0.125,-0.484254474936005,0.586834729715275));
#10027=CARTESIAN_POINT('Ctrl Pts',(-0.125,-0.5,0.586834729715275));
#10028=CARTESIAN_POINT('Ctrl Pts',(-0.125,-0.5,0.586834729715275));
#10029=CARTESIAN_POINT('Ctrl Pts',(-0.125,-0.515745525063995,0.586834729715275));
#10030=CARTESIAN_POINT('Ctrl Pts',(-0.121843784097853,-0.532507913768158,
0.587534197873268));
#10031=CARTESIAN_POINT('Ctrl Pts',(-0.109073016834181,-0.563290995658393,
0.590038488226116));
#10032=CARTESIAN_POINT('Ctrl Pts',(-0.0994608796208941,-0.577315815675743,
0.591804743154611));
#10033=CARTESIAN_POINT('Ctrl Pts',(-0.077316548567853,-0.599460146728784,
0.59510289473619));
#10034=CARTESIAN_POINT('Ctrl Pts',(-0.0632914182239687,-0.609072857638709,
0.596852269967858));
#10035=CARTESIAN_POINT('Ctrl Pts',(-0.0325072544867635,-0.621844041497889,
0.599317707212167));
#10036=CARTESIAN_POINT('Ctrl Pts',(-0.0157444828659572,-0.625,0.6));
#10037=CARTESIAN_POINT('Ctrl Pts',(0.0157444828659572,-0.625,0.6));
#10038=CARTESIAN_POINT('Ctrl Pts',(0.0325072544867633,-0.621844041497889,
0.599317707212167));
#10039=CARTESIAN_POINT('Ctrl Pts',(0.0632914182239686,-0.609072857638709,
0.596852269967858));
#10040=CARTESIAN_POINT('Ctrl Pts',(0.077316548567853,-0.599460146728784,
0.59510289473619));
#10041=CARTESIAN_POINT('Ctrl Pts',(0.0994608796208942,-0.577315815675743,
0.591804743154611));
#10042=CARTESIAN_POINT('Ctrl Pts',(0.109073016834181,-0.563290995658393,
0.590038488226116));
#10043=CARTESIAN_POINT('Ctrl Pts',(0.121843784097853,-0.532507913768158,
0.587534197873268));
#10044=CARTESIAN_POINT('Ctrl Pts',(0.125,-0.515745525063995,0.586834729715275));
#10045=CARTESIAN_POINT('Ctrl Pts',(0.125,-0.5,0.586834729715275));
#10046=CARTESIAN_POINT('',(-0.586834729715275,-0.5,-0.125));
#10047=CARTESIAN_POINT('',(-0.586834729715275,-0.5,0.125));
#10048=CARTESIAN_POINT('Ctrl Pts',(-0.586834729715275,-0.5,-0.125));
#10049=CARTESIAN_POINT('Ctrl Pts',(-0.586834729715275,-0.515745525063995,
-0.125));
#10050=CARTESIAN_POINT('Ctrl Pts',(-0.587534197873268,-0.532507913768158,
-0.121843784097853));
#10051=CARTESIAN_POINT('Ctrl Pts',(-0.590038488226116,-0.563290995658393,
-0.109073016834181));
#10052=CARTESIAN_POINT('Ctrl Pts',(-0.591804743154611,-0.577315815675743,
-0.0994608796208942));
#10053=CARTESIAN_POINT('Ctrl Pts',(-0.59510289473619,-0.599460146728784,
-0.0773165485678531));
#10054=CARTESIAN_POINT('Ctrl Pts',(-0.596852269967858,-0.609072857638709,
-0.0632914182239687));
#10055=CARTESIAN_POINT('Ctrl Pts',(-0.599317707212167,-0.621844041497889,
-0.0325072544867635));
#10056=CARTESIAN_POINT('Ctrl Pts',(-0.6,-0.625,-0.0157444828659573));
#10057=CARTESIAN_POINT('Ctrl Pts',(-0.6,-0.625,0.0157444828659572));
#10058=CARTESIAN_POINT('Ctrl Pts',(-0.599317707212167,-0.621844041497889,
0.0325072544867633));
#10059=CARTESIAN_POINT('Ctrl Pts',(-0.596852269967858,-0.609072857638709,
0.0632914182239686));
#10060=CARTESIAN_POINT('Ctrl Pts',(-0.59510289473619,-0.599460146728784,
0.077316548567853));
#10061=CARTESIAN_POINT('Ctrl Pts',(-0.591804743154611,-0.577315815675743,
0.0994608796208941));
#10062=CARTESIAN_POINT('Ctrl Pts',(-0.590038488226116,-0.563290995658393,
0.109073016834181));
#10063=CARTESIAN_POINT('Ctrl Pts',(-0.587534197873268,-0.532507913768158,
0.121843784097853));
#10064=CARTESIAN_POINT('Ctrl Pts',(-0.586834729715275,-0.515745525063995,
0.125));
#10065=CARTESIAN_POINT('Ctrl Pts',(-0.586834729715275,-0.5,0.125));
#10066=CARTESIAN_POINT('Ctrl Pts',(-0.586834729715275,-0.5,0.125));
#10067=CARTESIAN_POINT('Ctrl Pts',(-0.586834729715275,-0.484254474936005,
0.125));
#10068=CARTESIAN_POINT('Ctrl Pts',(-0.587534197873268,-0.467492086231842,
0.121843784097853));
#10069=CARTESIAN_POINT('Ctrl Pts',(-0.590038488226116,-0.436709004341607,
0.109073016834181));
#10070=CARTESIAN_POINT('Ctrl Pts',(-0.591804743154611,-0.422684184324257,
0.0994608796208941));
#10071=CARTESIAN_POINT('Ctrl Pts',(-0.59510289473619,-0.400539853271216,
0.077316548567853));
#10072=CARTESIAN_POINT('Ctrl Pts',(-0.596852269967858,-0.390927142361291,
0.0632914182239686));
#10073=CARTESIAN_POINT('Ctrl Pts',(-0.599317707212167,-0.378155958502111,
0.0325072544867634));
#10074=CARTESIAN_POINT('Ctrl Pts',(-0.6,-0.375,0.0157444828659572));
#10075=CARTESIAN_POINT('Ctrl Pts',(-0.6,-0.375,-0.0157444828659572));
#10076=CARTESIAN_POINT('Ctrl Pts',(-0.599317707212167,-0.378155958502111,
-0.0325072544867634));
#10077=CARTESIAN_POINT('Ctrl Pts',(-0.596852269967858,-0.390927142361291,
-0.0632914182239686));
#10078=CARTESIAN_POINT('Ctrl Pts',(-0.59510289473619,-0.400539853271216,
-0.077316548567853));
#10079=CARTESIAN_POINT('Ctrl Pts',(-0.591804743154611,-0.422684184324257,
-0.0994608796208942));
#10080=CARTESIAN_POINT('Ctrl Pts',(-0.590038488226116,-0.436709004341607,
-0.109073016834181));
#10081=CARTESIAN_POINT('Ctrl Pts',(-0.587534197873268,-0.467492086231842,
-0.121843784097853));
#10082=CARTESIAN_POINT('Ctrl Pts',(-0.586834729715275,-0.484254474936005,
-0.125));
#10083=CARTESIAN_POINT('Ctrl Pts',(-0.586834729715275,-0.5,-0.125));
#10084=CARTESIAN_POINT('',(0.586834729715275,-0.5,-0.125));
#10085=CARTESIAN_POINT('',(0.586834729715275,-0.5,0.125));
#10086=CARTESIAN_POINT('Ctrl Pts',(0.586834729715275,-0.5,-0.125));
#10087=CARTESIAN_POINT('Ctrl Pts',(0.586834729715275,-0.484254474936005,
-0.125));
#10088=CARTESIAN_POINT('Ctrl Pts',(0.587534197873268,-0.467492086231842,
-0.121843784097853));
#10089=CARTESIAN_POINT('Ctrl Pts',(0.590038488226116,-0.436709004341607,
-0.109073016834181));
#10090=CARTESIAN_POINT('Ctrl Pts',(0.591804743154611,-0.422684184324257,
-0.0994608796208941));
#10091=CARTESIAN_POINT('Ctrl Pts',(0.59510289473619,-0.400539853271216,
-0.0773165485678529));
#10092=CARTESIAN_POINT('Ctrl Pts',(0.596852269967858,-0.390927142361291,
-0.0632914182239686));
#10093=CARTESIAN_POINT('Ctrl Pts',(0.599317707212167,-0.378155958502111,
-0.0325072544867633));
#10094=CARTESIAN_POINT('Ctrl Pts',(0.6,-0.375,-0.0157444828659572));
#10095=CARTESIAN_POINT('Ctrl Pts',(0.6,-0.375,0.0157444828659573));
#10096=CARTESIAN_POINT('Ctrl Pts',(0.599317707212167,-0.378155958502111,
0.0325072544867635));
#10097=CARTESIAN_POINT('Ctrl Pts',(0.596852269967858,-0.390927142361291,
0.0632914182239687));
#10098=CARTESIAN_POINT('Ctrl Pts',(0.59510289473619,-0.400539853271216,
0.0773165485678531));
#10099=CARTESIAN_POINT('Ctrl Pts',(0.591804743154611,-0.422684184324257,
0.0994608796208942));
#10100=CARTESIAN_POINT('Ctrl Pts',(0.590038488226116,-0.436709004341607,
0.109073016834181));
#10101=CARTESIAN_POINT('Ctrl Pts',(0.587534197873268,-0.467492086231842,
0.121843784097853));
#10102=CARTESIAN_POINT('Ctrl Pts',(0.586834729715275,-0.484254474936005,
0.125));
#10103=CARTESIAN_POINT('Ctrl Pts',(0.586834729715275,-0.5,0.125));
#10104=CARTESIAN_POINT('Ctrl Pts',(0.586834729715275,-0.5,0.125));
#10105=CARTESIAN_POINT('Ctrl Pts',(0.586834729715275,-0.515745525063995,
0.125));
#10106=CARTESIAN_POINT('Ctrl Pts',(0.587534197873268,-0.532507913768158,
0.121843784097853));
#10107=CARTESIAN_POINT('Ctrl Pts',(0.590038488226116,-0.563290995658393,
0.109073016834181));
#10108=CARTESIAN_POINT('Ctrl Pts',(0.591804743154611,-0.577315815675743,
0.0994608796208942));
#10109=CARTESIAN_POINT('Ctrl Pts',(0.59510289473619,-0.599460146728784,
0.077316548567853));
#10110=CARTESIAN_POINT('Ctrl Pts',(0.596852269967858,-0.609072857638709,
0.0632914182239688));
#10111=CARTESIAN_POINT('Ctrl Pts',(0.599317707212167,-0.621844041497889,
0.0325072544867635));
#10112=CARTESIAN_POINT('Ctrl Pts',(0.6,-0.625,0.0157444828659573));
#10113=CARTESIAN_POINT('Ctrl Pts',(0.6,-0.625,-0.0157444828659572));
#10114=CARTESIAN_POINT('Ctrl Pts',(0.599317707212167,-0.621844041497889,
-0.0325072544867633));
#10115=CARTESIAN_POINT('Ctrl Pts',(0.596852269967858,-0.609072857638709,
-0.0632914182239685));
#10116=CARTESIAN_POINT('Ctrl Pts',(0.59510289473619,-0.599460146728784,
-0.077316548567853));
#10117=CARTESIAN_POINT('Ctrl Pts',(0.591804743154611,-0.577315815675743,
-0.0994608796208941));
#10118=CARTESIAN_POINT('Ctrl Pts',(0.590038488226116,-0.563290995658393,
-0.10907301683418));
#10119=CARTESIAN_POINT('Ctrl Pts',(0.587534197873268,-0.532507913768158,
-0.121843784097853));
#10120=CARTESIAN_POINT('Ctrl Pts',(0.586834729715275,-0.515745525063995,
-0.125));
#10121=CARTESIAN_POINT('Ctrl Pts',(0.586834729715275,-0.5,-0.125));
#10122=CARTESIAN_POINT('Origin',(0.,-0.5,0.));
#10123=CARTESIAN_POINT('',(-1.,-0.375,-6.12323399573677E-17));
#10124=CARTESIAN_POINT('',(-0.992156741649222,-0.5,0.125));
#10125=CARTESIAN_POINT('Ctrl Pts',(-1.,-0.375,-1.00613961606655E-16));
#10126=CARTESIAN_POINT('Ctrl Pts',(-1.,-0.375,0.0157128711428661));
#10127=CARTESIAN_POINT('Ctrl Pts',(-0.999591823858855,-0.378143583103513,
0.0324619190698278));
#10128=CARTESIAN_POINT('Ctrl Pts',(-0.998116453123232,-0.390905426591754,
0.0632545375991437));
#10129=CARTESIAN_POINT('Ctrl Pts',(-0.997070068816062,-0.400522781657727,
0.0772994769543643));
#10130=CARTESIAN_POINT('Ctrl Pts',(-0.995102104277285,-0.422700615683787,
0.0994773109804239));
#10131=CARTESIAN_POINT('Ctrl Pts',(-0.994052129228928,-0.436745514765346,
0.109094593469654));
#10132=CARTESIAN_POINT('Ctrl Pts',(-0.99256853061881,-0.467537996927464,
0.121856383722779));
#10133=CARTESIAN_POINT('Ctrl Pts',(-0.992156741649222,-0.484286997589363,
0.125));
#10134=CARTESIAN_POINT('Ctrl Pts',(-0.992156741649222,-0.5,0.125));
#10135=CARTESIAN_POINT('',(-1.,-0.625,-6.12323399573677E-17));
#10136=CARTESIAN_POINT('Ctrl Pts',(-1.,-0.625,-4.5102810375397E-17));
#10137=CARTESIAN_POINT('Ctrl Pts',(-1.,-0.625,-0.0157128711428662));
#10138=CARTESIAN_POINT('Ctrl Pts',(-0.999591823858855,-0.621856416896487,
-0.032461919069828));
#10139=CARTESIAN_POINT('Ctrl Pts',(-0.998116453123232,-0.609094573408246,
-0.0632545375991439));
#10140=CARTESIAN_POINT('Ctrl Pts',(-0.997070068816062,-0.599477218342273,
-0.0772994769543645));
#10141=CARTESIAN_POINT('Ctrl Pts',(-0.995102104277285,-0.577299384316213,
-0.0994773109804241));
#10142=CARTESIAN_POINT('Ctrl Pts',(-0.994052129228928,-0.563254485234654,
-0.109094593469655));
#10143=CARTESIAN_POINT('Ctrl Pts',(-0.99256853061881,-0.532462003072536,
-0.121856383722779));
#10144=CARTESIAN_POINT('Ctrl Pts',(-0.992156741649221,-0.515713002410637,
-0.125));
#10145=CARTESIAN_POINT('Ctrl Pts',(-0.992156741649221,-0.484286997589363,
-0.125));
#10146=CARTESIAN_POINT('Ctrl Pts',(-0.99256853061881,-0.467537996927464,
-0.121856383722779));
#10147=CARTESIAN_POINT('Ctrl Pts',(-0.994052129228928,-0.436745514765346,
-0.109094593469655));
#10148=CARTESIAN_POINT('Ctrl Pts',(-0.995102104277285,-0.422700615683787,
-0.0994773109804241));
#10149=CARTESIAN_POINT('Ctrl Pts',(-0.997070068816062,-0.400522781657728,
-0.0772994769543645));
#10150=CARTESIAN_POINT('Ctrl Pts',(-0.998116453123232,-0.390905426591754,
-0.063254537599144));
#10151=CARTESIAN_POINT('Ctrl Pts',(-0.999591823858855,-0.378143583103513,
-0.0324619190698281));
#10152=CARTESIAN_POINT('Ctrl Pts',(-1.,-0.375,-0.0157128711428663));
#10153=CARTESIAN_POINT('Ctrl Pts',(-1.,-0.375,-9.36750677027476E-17));
#10154=CARTESIAN_POINT('Ctrl Pts',(-0.992156741649222,-0.5,0.125));
#10155=CARTESIAN_POINT('Ctrl Pts',(-0.992156741649222,-0.515713002410637,
0.125));
#10156=CARTESIAN_POINT('Ctrl Pts',(-0.99256853061881,-0.532462003072536,
0.121856383722779));
#10157=CARTESIAN_POINT('Ctrl Pts',(-0.994052129228928,-0.563254485234654,
0.109094593469654));
#10158=CARTESIAN_POINT('Ctrl Pts',(-0.995102104277285,-0.577299384316213,
0.0994773109804241));
#10159=CARTESIAN_POINT('Ctrl Pts',(-0.997070068816062,-0.599477218342273,
0.0772994769543644));
#10160=CARTESIAN_POINT('Ctrl Pts',(-0.998116453123232,-0.609094573408246,
0.0632545375991438));
#10161=CARTESIAN_POINT('Ctrl Pts',(-0.999591823858855,-0.621856416896487,
0.0324619190698279));
#10162=CARTESIAN_POINT('Ctrl Pts',(-1.,-0.625,0.0157128711428661));
#10163=CARTESIAN_POINT('Ctrl Pts',(-1.,-0.625,-4.85722573273506E-17));
#10164=CARTESIAN_POINT('',(-7.65404249467096E-18,-0.5,0.125));
#10165=CARTESIAN_POINT('Origin',(0.,-0.5,0.));
#10166=CARTESIAN_POINT('',(0.992156741649222,-0.5,0.125));
#10167=CARTESIAN_POINT('',(-7.65404249467096E-18,-0.5,0.125));
#10168=CARTESIAN_POINT('',(1.,-0.625,6.12323399573677E-17));
#10169=CARTESIAN_POINT('Ctrl Pts',(1.,-0.625,7.28583859910259E-17));
#10170=CARTESIAN_POINT('Ctrl Pts',(1.,-0.625,0.0157128711428663));
#10171=CARTESIAN_POINT('Ctrl Pts',(0.999591823858855,-0.621856416896487,
0.032461919069828));
#10172=CARTESIAN_POINT('Ctrl Pts',(0.998116453123232,-0.609094573408246,
0.0632545375991439));
#10173=CARTESIAN_POINT('Ctrl Pts',(0.997070068816062,-0.599477218342273,
0.0772994769543645));
#10174=CARTESIAN_POINT('Ctrl Pts',(0.995102104277285,-0.577299384316213,
0.0994773109804242));
#10175=CARTESIAN_POINT('Ctrl Pts',(0.994052129228928,-0.563254485234654,
0.109094593469655));
#10176=CARTESIAN_POINT('Ctrl Pts',(0.99256853061881,-0.532462003072536,
0.121856383722779));
#10177=CARTESIAN_POINT('Ctrl Pts',(0.992156741649222,-0.515713002410637,
0.125));
#10178=CARTESIAN_POINT('Ctrl Pts',(0.992156741649222,-0.5,0.125));
#10179=CARTESIAN_POINT('',(1.,-0.375,6.12323399573677E-17));
#10180=CARTESIAN_POINT('Ctrl Pts',(1.,-0.375,2.08166817117217E-17));
#10181=CARTESIAN_POINT('Ctrl Pts',(1.,-0.375,-0.0157128711428662));
#10182=CARTESIAN_POINT('Ctrl Pts',(0.999591823858855,-0.378143583103513,
-0.032461919069828));
#10183=CARTESIAN_POINT('Ctrl Pts',(0.998116453123232,-0.390905426591754,
-0.0632545375991438));
#10184=CARTESIAN_POINT('Ctrl Pts',(0.997070068816062,-0.400522781657728,
-0.0772994769543644));
#10185=CARTESIAN_POINT('Ctrl Pts',(0.995102104277285,-0.422700615683787,
-0.099477310980424));
#10186=CARTESIAN_POINT('Ctrl Pts',(0.994052129228928,-0.436745514765346,
-0.109094593469654));
#10187=CARTESIAN_POINT('Ctrl Pts',(0.99256853061881,-0.467537996927464,
-0.121856383722779));
#10188=CARTESIAN_POINT('Ctrl Pts',(0.992156741649222,-0.484286997589363,
-0.125));
#10189=CARTESIAN_POINT('Ctrl Pts',(0.992156741649222,-0.515713002410637,
-0.125));
#10190=CARTESIAN_POINT('Ctrl Pts',(0.99256853061881,-0.532462003072536,
-0.121856383722779));
#10191=CARTESIAN_POINT('Ctrl Pts',(0.994052129228928,-0.563254485234654,
-0.109094593469654));
#10192=CARTESIAN_POINT('Ctrl Pts',(0.995102104277285,-0.577299384316213,
-0.099477310980424));
#10193=CARTESIAN_POINT('Ctrl Pts',(0.997070068816062,-0.599477218342273,
-0.0772994769543643));
#10194=CARTESIAN_POINT('Ctrl Pts',(0.998116453123232,-0.609094573408246,
-0.0632545375991438));
#10195=CARTESIAN_POINT('Ctrl Pts',(0.999591823858855,-0.621856416896487,
-0.0324619190698279));
#10196=CARTESIAN_POINT('Ctrl Pts',(1.,-0.625,-0.0157128711428661));
#10197=CARTESIAN_POINT('Ctrl Pts',(1.,-0.625,8.32667268468867E-17));
#10198=CARTESIAN_POINT('Ctrl Pts',(0.992156741649222,-0.5,0.125));
#10199=CARTESIAN_POINT('Ctrl Pts',(0.992156741649222,-0.484286997589363,
0.125));
#10200=CARTESIAN_POINT('Ctrl Pts',(0.99256853061881,-0.467537996927464,
0.121856383722779));
#10201=CARTESIAN_POINT('Ctrl Pts',(0.994052129228928,-0.436745514765346,
0.109094593469654));
#10202=CARTESIAN_POINT('Ctrl Pts',(0.995102104277285,-0.422700615683787,
0.0994773109804241));
#10203=CARTESIAN_POINT('Ctrl Pts',(0.997070068816062,-0.400522781657727,
0.0772994769543644));
#10204=CARTESIAN_POINT('Ctrl Pts',(0.998116453123232,-0.390905426591754,
0.0632545375991438));
#10205=CARTESIAN_POINT('Ctrl Pts',(0.999591823858855,-0.378143583103513,
0.0324619190698279));
#10206=CARTESIAN_POINT('Ctrl Pts',(1.,-0.375,0.0157128711428662));
#10207=CARTESIAN_POINT('Ctrl Pts',(1.,-0.375,2.77555756156289E-17));
#10208=CARTESIAN_POINT('Origin',(0.,-0.1,0.));
#10209=CARTESIAN_POINT('',(-1.,-0.9,1.22464679914735E-16));
#10210=CARTESIAN_POINT('Origin',(0.,-0.9,0.));
#10211=CARTESIAN_POINT('',(-1.,-0.1,-1.22464679914735E-16));
#10212=CARTESIAN_POINT('',(-1.,-0.1,1.22464679914735E-16));
#10213=CARTESIAN_POINT('',(-1.,-0.1,-1.22464679914735E-16));
#10214=CARTESIAN_POINT('Origin',(0.,-0.1,0.));
#10215=CARTESIAN_POINT('',(0.,-0.625,-1.));
#10216=CARTESIAN_POINT('',(0.,-0.375,-1.));
#10217=CARTESIAN_POINT('Ctrl Pts',(-2.08166817117217E-17,-0.625,-1.));
#10218=CARTESIAN_POINT('Ctrl Pts',(0.0157128711428662,-0.625,-1.));
#10219=CARTESIAN_POINT('Ctrl Pts',(0.0324619190698279,-0.621856416896487,
-0.999591823858855));
#10220=CARTESIAN_POINT('Ctrl Pts',(0.0632545375991438,-0.609094573408246,
-0.998116453123232));
#10221=CARTESIAN_POINT('Ctrl Pts',(0.0772994769543644,-0.599477218342273,
-0.997070068816062));
#10222=CARTESIAN_POINT('Ctrl Pts',(0.0994773109804241,-0.577299384316213,
-0.995102104277285));
#10223=CARTESIAN_POINT('Ctrl Pts',(0.109094593469654,-0.563254485234654,
-0.994052129228928));
#10224=CARTESIAN_POINT('Ctrl Pts',(0.121856383722779,-0.532462003072536,
-0.99256853061881));
#10225=CARTESIAN_POINT('Ctrl Pts',(0.125,-0.515713002410637,-0.992156741649221));
#10226=CARTESIAN_POINT('Ctrl Pts',(0.125,-0.484286997589363,-0.992156741649221));
#10227=CARTESIAN_POINT('Ctrl Pts',(0.121856383722779,-0.467537996927464,
-0.99256853061881));
#10228=CARTESIAN_POINT('Ctrl Pts',(0.109094593469654,-0.436745514765346,
-0.994052129228928));
#10229=CARTESIAN_POINT('Ctrl Pts',(0.0994773109804241,-0.422700615683787,
-0.995102104277285));
#10230=CARTESIAN_POINT('Ctrl Pts',(0.0772994769543645,-0.400522781657728,
-0.997070068816062));
#10231=CARTESIAN_POINT('Ctrl Pts',(0.0632545375991439,-0.390905426591754,
-0.998116453123232));
#10232=CARTESIAN_POINT('Ctrl Pts',(0.032461919069828,-0.378143583103513,
-0.999591823858855));
#10233=CARTESIAN_POINT('Ctrl Pts',(0.0157128711428662,-0.375,-1.));
#10234=CARTESIAN_POINT('Ctrl Pts',(3.81639164714898E-17,-0.375,-1.));
#10235=CARTESIAN_POINT('',(-0.125,-0.5,-0.992156741649222));
#10236=CARTESIAN_POINT('Ctrl Pts',(4.5102810375397E-17,-0.375,-1.));
#10237=CARTESIAN_POINT('Ctrl Pts',(-0.0157128711428661,-0.375,-1.));
#10238=CARTESIAN_POINT('Ctrl Pts',(-0.0324619190698279,-0.378143583103513,
-0.999591823858855));
#10239=CARTESIAN_POINT('Ctrl Pts',(-0.0632545375991437,-0.390905426591754,
-0.998116453123232));
#10240=CARTESIAN_POINT('Ctrl Pts',(-0.0772994769543643,-0.400522781657727,
-0.997070068816062));
#10241=CARTESIAN_POINT('Ctrl Pts',(-0.099477310980424,-0.422700615683787,
-0.995102104277285));
#10242=CARTESIAN_POINT('Ctrl Pts',(-0.109094593469654,-0.436745514765346,
-0.994052129228928));
#10243=CARTESIAN_POINT('Ctrl Pts',(-0.121856383722779,-0.467537996927464,
-0.99256853061881));
#10244=CARTESIAN_POINT('Ctrl Pts',(-0.125,-0.484286997589363,-0.992156741649222));
#10245=CARTESIAN_POINT('Ctrl Pts',(-0.125,-0.5,-0.992156741649222));
#10246=CARTESIAN_POINT('Ctrl Pts',(-0.125,-0.5,-0.992156741649222));
#10247=CARTESIAN_POINT('Ctrl Pts',(-0.125,-0.515713002410637,-0.992156741649222));
#10248=CARTESIAN_POINT('Ctrl Pts',(-0.121856383722779,-0.532462003072536,
-0.99256853061881));
#10249=CARTESIAN_POINT('Ctrl Pts',(-0.109094593469654,-0.563254485234654,
-0.994052129228928));
#10250=CARTESIAN_POINT('Ctrl Pts',(-0.0994773109804241,-0.577299384316213,
-0.995102104277285));
#10251=CARTESIAN_POINT('Ctrl Pts',(-0.0772994769543644,-0.599477218342273,
-0.997070068816062));
#10252=CARTESIAN_POINT('Ctrl Pts',(-0.0632545375991439,-0.609094573408246,
-0.998116453123232));
#10253=CARTESIAN_POINT('Ctrl Pts',(-0.032461919069828,-0.621856416896487,
-0.999591823858855));
#10254=CARTESIAN_POINT('Ctrl Pts',(-0.0157128711428662,-0.625,-1.));
#10255=CARTESIAN_POINT('Ctrl Pts',(-1.38777878078145E-17,-0.625,-1.));
#10256=CARTESIAN_POINT('',(0.,-0.375,1.));
#10257=CARTESIAN_POINT('',(0.,-0.625,1.));
#10258=CARTESIAN_POINT('Ctrl Pts',(4.16333634234434E-17,-0.375,1.));
#10259=CARTESIAN_POINT('Ctrl Pts',(0.0157128711428662,-0.375,1.));
#10260=CARTESIAN_POINT('Ctrl Pts',(0.032461919069828,-0.378143583103513,
0.999591823858855));
#10261=CARTESIAN_POINT('Ctrl Pts',(0.0632545375991439,-0.390905426591754,
0.998116453123232));
#10262=CARTESIAN_POINT('Ctrl Pts',(0.0772994769543644,-0.400522781657728,
0.997070068816062));
#10263=CARTESIAN_POINT('Ctrl Pts',(0.0994773109804241,-0.422700615683787,
0.995102104277285));
#10264=CARTESIAN_POINT('Ctrl Pts',(0.109094593469654,-0.436745514765346,
0.994052129228928));
#10265=CARTESIAN_POINT('Ctrl Pts',(0.121856383722779,-0.467537996927464,
0.99256853061881));
#10266=CARTESIAN_POINT('Ctrl Pts',(0.125,-0.484286997589363,0.992156741649222));
#10267=CARTESIAN_POINT('Ctrl Pts',(0.125,-0.515713002410637,0.992156741649222));
#10268=CARTESIAN_POINT('Ctrl Pts',(0.121856383722779,-0.532462003072536,
0.99256853061881));
#10269=CARTESIAN_POINT('Ctrl Pts',(0.109094593469655,-0.563254485234654,
0.994052129228928));
#10270=CARTESIAN_POINT('Ctrl Pts',(0.0994773109804241,-0.577299384316213,
0.995102104277285));
#10271=CARTESIAN_POINT('Ctrl Pts',(0.0772994769543644,-0.599477218342273,
0.997070068816062));
#10272=CARTESIAN_POINT('Ctrl Pts',(0.0632545375991438,-0.609094573408246,
0.998116453123232));
#10273=CARTESIAN_POINT('Ctrl Pts',(0.0324619190698279,-0.621856416896487,
0.999591823858855));
#10274=CARTESIAN_POINT('Ctrl Pts',(0.0157128711428662,-0.625,1.));
#10275=CARTESIAN_POINT('Ctrl Pts',(-1.73472347597681E-17,-0.625,1.));
#10276=CARTESIAN_POINT('',(-0.125,-0.5,0.992156741649222));
#10277=CARTESIAN_POINT('Ctrl Pts',(-1.73472347597681E-17,-0.625,1.));
#10278=CARTESIAN_POINT('Ctrl Pts',(-0.0157128711428662,-0.625,1.));
#10279=CARTESIAN_POINT('Ctrl Pts',(-0.032461919069828,-0.621856416896487,
0.999591823858855));
#10280=CARTESIAN_POINT('Ctrl Pts',(-0.0632545375991439,-0.609094573408246,
0.998116453123232));
#10281=CARTESIAN_POINT('Ctrl Pts',(-0.0772994769543645,-0.599477218342273,
0.997070068816062));
#10282=CARTESIAN_POINT('Ctrl Pts',(-0.0994773109804241,-0.577299384316213,
0.995102104277285));
#10283=CARTESIAN_POINT('Ctrl Pts',(-0.109094593469654,-0.563254485234654,
0.994052129228928));
#10284=CARTESIAN_POINT('Ctrl Pts',(-0.121856383722779,-0.532462003072536,
0.99256853061881));
#10285=CARTESIAN_POINT('Ctrl Pts',(-0.125,-0.515713002410637,0.992156741649222));
#10286=CARTESIAN_POINT('Ctrl Pts',(-0.125,-0.5,0.992156741649222));
#10287=CARTESIAN_POINT('Ctrl Pts',(-0.125,-0.5,0.992156741649222));
#10288=CARTESIAN_POINT('Ctrl Pts',(-0.125,-0.484286997589363,0.992156741649222));
#10289=CARTESIAN_POINT('Ctrl Pts',(-0.121856383722779,-0.467537996927464,
0.99256853061881));
#10290=CARTESIAN_POINT('Ctrl Pts',(-0.109094593469654,-0.436745514765346,
0.994052129228928));
#10291=CARTESIAN_POINT('Ctrl Pts',(-0.099477310980424,-0.422700615683787,
0.995102104277285));
#10292=CARTESIAN_POINT('Ctrl Pts',(-0.0772994769543643,-0.400522781657727,
0.997070068816062));
#10293=CARTESIAN_POINT('Ctrl Pts',(-0.0632545375991438,-0.390905426591754,
0.998116453123232));
#10294=CARTESIAN_POINT('Ctrl Pts',(-0.0324619190698279,-0.378143583103513,
0.999591823858855));
#10295=CARTESIAN_POINT('Ctrl Pts',(-0.0157128711428661,-0.375,1.));
#10296=CARTESIAN_POINT('Ctrl Pts',(4.5102810375397E-17,-0.375,1.));
#10297=CARTESIAN_POINT('Origin',(0.,-0.5,0.));
#10298=CARTESIAN_POINT('',(-0.125,-0.5,0.));
#10299=CARTESIAN_POINT('Origin',(0.,-0.5,0.));
#10300=CARTESIAN_POINT('',(-0.125,-0.5,0.));
#10301=CARTESIAN_POINT('Origin',(0.,-0.9,0.));
#10302=CARTESIAN_POINT('Origin',(0.,0.,0.));
#10303=CARTESIAN_POINT('',(-1.4,0.,1.71450551880629E-16));
#10304=CARTESIAN_POINT('Origin',(0.,0.,0.));
#10305=CARTESIAN_POINT('',(1.23958209161204,0.,0.143317017690053));
#10306=CARTESIAN_POINT('',(1.22320001975977,0.,0.246749348660852));
#10307=CARTESIAN_POINT('Origin',(1.21321664662686,0.,0.192154639568406));
#10308=CARTESIAN_POINT('',(1.20190105810224,0.,0.335465908756113));
#10309=CARTESIAN_POINT('Origin',(0.,0.,0.));
#10310=CARTESIAN_POINT('',(1.16954029537568,0.,0.435062095450087));
#10311=CARTESIAN_POINT('Origin',(1.1682203282434,0.,0.379577794185952));
#10312=CARTESIAN_POINT('',(1.13462523166105,0.,0.519354515801077));
#10313=CARTESIAN_POINT('Origin',(0.,0.,0.));
#10314=CARTESIAN_POINT('',(1.08708260743774,0.,0.612662169561029));
#10315=CARTESIAN_POINT('Origin',(1.0944585482776,0.,0.557654483764164));
#10316=CARTESIAN_POINT('',(1.0394111664111,0.,0.690454891028201));
#10317=CARTESIAN_POINT('Origin',(0.,0.,0.));
#10318=CARTESIAN_POINT('',(0.977857337884349,0.,0.775176467748211));
#10319=CARTESIAN_POINT('Origin',(0.993747566553533,0.,0.72199986920298));
#10320=CARTESIAN_POINT('',(0.918603348636233,0.,0.844553975349804));
#10321=CARTESIAN_POINT('Origin',(0.,0.,0.));
#10322=CARTESIAN_POINT('',(0.844553975349804,0.,0.918603348636233));
#10323=CARTESIAN_POINT('Origin',(0.86856722168183,0.,0.86856722168183));
#10324=CARTESIAN_POINT('',(0.775176467748211,0.,0.977857337884349));
#10325=CARTESIAN_POINT('Origin',(0.,0.,0.));
#10326=CARTESIAN_POINT('',(0.690454891028201,0.,1.0394111664111));
#10327=CARTESIAN_POINT('Origin',(0.721999869202979,0.,0.993747566553533));
#10328=CARTESIAN_POINT('',(0.612662169561028,0.,1.08708260743774));
#10329=CARTESIAN_POINT('Origin',(0.,0.,0.));
#10330=CARTESIAN_POINT('',(0.519354515801077,0.,1.13462523166105));
#10331=CARTESIAN_POINT('Origin',(0.557654483764164,0.,1.0944585482776));
#10332=CARTESIAN_POINT('',(0.435062095450087,0.,1.16954029537568));
#10333=CARTESIAN_POINT('Origin',(0.,0.,0.));
#10334=CARTESIAN_POINT('',(0.335465908756113,0.,1.20190105810224));
#10335=CARTESIAN_POINT('Origin',(0.379577794185951,0.,1.1682203282434));
#10336=CARTESIAN_POINT('',(0.246749348660851,0.,1.22320001975977));
#10337=CARTESIAN_POINT('Origin',(0.,0.,0.));
#10338=CARTESIAN_POINT('',(0.143317017690053,0.,1.23958209161204));
#10339=CARTESIAN_POINT('Origin',(0.192154639568406,0.,1.21321664662686));
#10340=CARTESIAN_POINT('',(0.0523608139934478,0.,1.24674050008925));
#10341=CARTESIAN_POINT('Origin',(0.,0.,0.));
#10342=CARTESIAN_POINT('',(-0.0523608139934483,0.,1.24674050008925));
#10343=CARTESIAN_POINT('Origin',(-2.25642313758905E-16,0.,1.22833954473516));
#10344=CARTESIAN_POINT('',(-0.143317017690053,0.,1.23958209161204));
#10345=CARTESIAN_POINT('Origin',(0.,0.,0.));
#10346=CARTESIAN_POINT('',(-0.246749348660852,0.,1.22320001975977));
#10347=CARTESIAN_POINT('Origin',(-0.192154639568406,0.,1.21321664662686));
#10348=CARTESIAN_POINT('',(-0.335465908756113,0.,1.20190105810224));
#10349=CARTESIAN_POINT('Origin',(0.,0.,0.));
#10350=CARTESIAN_POINT('',(-0.435062095450087,0.,1.16954029537568));
#10351=CARTESIAN_POINT('Origin',(-0.379577794185951,0.,1.1682203282434));
#10352=CARTESIAN_POINT('',(-0.519354515801077,0.,1.13462523166105));
#10353=CARTESIAN_POINT('Origin',(0.,0.,0.));
#10354=CARTESIAN_POINT('',(-0.612662169561029,0.,1.08708260743774));
#10355=CARTESIAN_POINT('Origin',(-0.557654483764164,0.,1.0944585482776));
#10356=CARTESIAN_POINT('',(-0.690454891028201,0.,1.0394111664111));
#10357=CARTESIAN_POINT('Origin',(0.,0.,0.));
#10358=CARTESIAN_POINT('',(-0.775176467748211,0.,0.977857337884349));
#10359=CARTESIAN_POINT('Origin',(-0.721999869202979,0.,0.993747566553533));
#10360=CARTESIAN_POINT('',(-0.844553975349804,0.,0.918603348636233));
#10361=CARTESIAN_POINT('Origin',(0.,0.,0.));
#10362=CARTESIAN_POINT('',(-0.918603348636233,0.,0.844553975349804));
#10363=CARTESIAN_POINT('Origin',(-0.86856722168183,0.,0.86856722168183));
#10364=CARTESIAN_POINT('',(-0.977857337884348,0.,0.775176467748211));
#10365=CARTESIAN_POINT('Origin',(0.,0.,0.));
#10366=CARTESIAN_POINT('',(-1.0394111664111,0.,0.690454891028201));
#10367=CARTESIAN_POINT('Origin',(-0.993747566553533,0.,0.721999869202979));
#10368=CARTESIAN_POINT('',(-1.08708260743774,0.,0.612662169561028));
#10369=CARTESIAN_POINT('Origin',(0.,0.,0.));
#10370=CARTESIAN_POINT('',(-1.13462523166105,0.,0.519354515801077));
#10371=CARTESIAN_POINT('Origin',(-1.0944585482776,0.,0.557654483764164));
#10372=CARTESIAN_POINT('',(-1.16954029537568,0.,0.435062095450087));
#10373=CARTESIAN_POINT('Origin',(0.,0.,0.));
#10374=CARTESIAN_POINT('',(-1.20190105810224,0.,0.335465908756113));
#10375=CARTESIAN_POINT('Origin',(-1.1682203282434,0.,0.379577794185951));
#10376=CARTESIAN_POINT('',(-1.22320001975977,0.,0.246749348660851));
#10377=CARTESIAN_POINT('Origin',(0.,0.,0.));
#10378=CARTESIAN_POINT('',(-1.23958209161204,0.,0.143317017690053));
#10379=CARTESIAN_POINT('Origin',(-1.21321664662686,0.,0.192154639568406));
#10380=CARTESIAN_POINT('',(-1.24674050008925,0.,0.0523608139934479));
#10381=CARTESIAN_POINT('Origin',(0.,0.,0.));
#10382=CARTESIAN_POINT('',(-1.24674050008925,0.,-0.0523608139934482));
#10383=CARTESIAN_POINT('Origin',(-1.22833954473516,0.,-1.50428209172603E-16));
#10384=CARTESIAN_POINT('',(-1.23958209161204,0.,-0.143317017690053));
#10385=CARTESIAN_POINT('Origin',(0.,0.,0.));
#10386=CARTESIAN_POINT('',(-1.22320001975977,0.,-0.246749348660852));
#10387=CARTESIAN_POINT('Origin',(-1.21321664662686,0.,-0.192154639568406));
#10388=CARTESIAN_POINT('',(-1.20190105810224,0.,-0.335465908756113));
#10389=CARTESIAN_POINT('Origin',(0.,0.,0.));
#10390=CARTESIAN_POINT('',(-1.16954029537568,0.,-0.435062095450087));
#10391=CARTESIAN_POINT('Origin',(-1.1682203282434,0.,-0.379577794185951));
#10392=CARTESIAN_POINT('',(-1.13462523166105,0.,-0.519354515801077));
#10393=CARTESIAN_POINT('Origin',(0.,0.,0.));
#10394=CARTESIAN_POINT('',(-1.08708260743774,0.,-0.612662169561029));
#10395=CARTESIAN_POINT('Origin',(-1.0944585482776,0.,-0.557654483764164));
#10396=CARTESIAN_POINT('',(-1.0394111664111,0.,-0.690454891028201));
#10397=CARTESIAN_POINT('Origin',(0.,0.,0.));
#10398=CARTESIAN_POINT('',(-0.977857337884349,0.,-0.775176467748211));
#10399=CARTESIAN_POINT('Origin',(-0.993747566553533,0.,-0.721999869202979));
#10400=CARTESIAN_POINT('',(-0.918603348636233,0.,-0.844553975349804));
#10401=CARTESIAN_POINT('Origin',(0.,0.,0.));
#10402=CARTESIAN_POINT('',(-0.844553975349804,0.,-0.918603348636233));
#10403=CARTESIAN_POINT('Origin',(-0.86856722168183,0.,-0.86856722168183));
#10404=CARTESIAN_POINT('',(-0.775176467748211,0.,-0.977857337884348));
#10405=CARTESIAN_POINT('Origin',(0.,0.,0.));
#10406=CARTESIAN_POINT('',(-0.690454891028201,0.,-1.0394111664111));
#10407=CARTESIAN_POINT('Origin',(-0.721999869202979,0.,-0.993747566553533));
#10408=CARTESIAN_POINT('',(-0.612662169561028,0.,-1.08708260743774));
#10409=CARTESIAN_POINT('Origin',(0.,0.,0.));
#10410=CARTESIAN_POINT('',(-0.519354515801077,0.,-1.13462523166105));
#10411=CARTESIAN_POINT('Origin',(-0.557654483764164,0.,-1.0944585482776));
#10412=CARTESIAN_POINT('',(-0.435062095450087,0.,-1.16954029537568));
#10413=CARTESIAN_POINT('Origin',(0.,0.,0.));
#10414=CARTESIAN_POINT('',(-0.335465908756113,0.,-1.20190105810224));
#10415=CARTESIAN_POINT('Origin',(-0.379577794185951,0.,-1.1682203282434));
#10416=CARTESIAN_POINT('',(-0.246749348660852,0.,-1.22320001975977));
#10417=CARTESIAN_POINT('Origin',(0.,0.,0.));
#10418=CARTESIAN_POINT('',(-0.143317017690053,0.,-1.23958209161204));
#10419=CARTESIAN_POINT('Origin',(-0.192154639568406,0.,-1.21321664662686));
#10420=CARTESIAN_POINT('',(-0.0523608139934479,0.,-1.24674050008925));
#10421=CARTESIAN_POINT('Origin',(0.,0.,0.));
#10422=CARTESIAN_POINT('',(0.0523608139934481,0.,-1.24674050008925));
#10423=CARTESIAN_POINT('Origin',(7.52141045863017E-17,0.,-1.22833954473516));
#10424=CARTESIAN_POINT('',(0.143317017690053,0.,-1.23958209161204));
#10425=CARTESIAN_POINT('Origin',(0.,0.,0.));
#10426=CARTESIAN_POINT('',(0.246749348660852,0.,-1.22320001975977));
#10427=CARTESIAN_POINT('Origin',(0.192154639568406,0.,-1.21321664662686));
#10428=CARTESIAN_POINT('',(0.335465908756113,0.,-1.20190105810224));
#10429=CARTESIAN_POINT('Origin',(0.,0.,0.));
#10430=CARTESIAN_POINT('',(0.435062095450087,0.,-1.16954029537568));
#10431=CARTESIAN_POINT('Origin',(0.379577794185951,0.,-1.1682203282434));
#10432=CARTESIAN_POINT('',(0.519354515801077,0.,-1.13462523166105));
#10433=CARTESIAN_POINT('Origin',(0.,0.,0.));
#10434=CARTESIAN_POINT('',(0.612662169561028,0.,-1.08708260743774));
#10435=CARTESIAN_POINT('Origin',(0.557654483764164,0.,-1.0944585482776));
#10436=CARTESIAN_POINT('',(0.690454891028201,0.,-1.0394111664111));
#10437=CARTESIAN_POINT('Origin',(0.,0.,0.));
#10438=CARTESIAN_POINT('',(0.775176467748211,0.,-0.977857337884349));
#10439=CARTESIAN_POINT('Origin',(0.721999869202979,0.,-0.993747566553533));
#10440=CARTESIAN_POINT('',(0.844553975349804,0.,-0.918603348636233));
#10441=CARTESIAN_POINT('Origin',(0.,0.,0.));
#10442=CARTESIAN_POINT('',(0.918603348636233,0.,-0.844553975349804));
#10443=CARTESIAN_POINT('Origin',(0.86856722168183,0.,-0.86856722168183));
#10444=CARTESIAN_POINT('',(0.977857337884349,0.,-0.775176467748211));
#10445=CARTESIAN_POINT('Origin',(0.,0.,0.));
#10446=CARTESIAN_POINT('',(1.0394111664111,0.,-0.690454891028201));
#10447=CARTESIAN_POINT('Origin',(0.993747566553533,0.,-0.721999869202979));
#10448=CARTESIAN_POINT('',(1.08708260743774,0.,-0.612662169561028));
#10449=CARTESIAN_POINT('Origin',(0.,0.,0.));
#10450=CARTESIAN_POINT('',(1.13462523166105,0.,-0.519354515801077));
#10451=CARTESIAN_POINT('Origin',(1.0944585482776,0.,-0.557654483764164));
#10452=CARTESIAN_POINT('',(1.16954029537568,0.,-0.43506209545009));
#10453=CARTESIAN_POINT('Origin',(0.,0.,0.));
#10454=CARTESIAN_POINT('',(1.20190105810224,0.,-0.33546590875611));
#10455=CARTESIAN_POINT('Origin',(1.1682203282434,0.,-0.379577794185951));
#10456=CARTESIAN_POINT('',(1.22320001975977,0.,-0.246749348660852));
#10457=CARTESIAN_POINT('Origin',(0.,0.,0.));
#10458=CARTESIAN_POINT('',(1.23958209161204,0.,-0.143317017690053));
#10459=CARTESIAN_POINT('Origin',(1.21321664662686,0.,-0.192154639568406));
#10460=CARTESIAN_POINT('',(1.24674050008925,0.,-0.052360813993451));
#10461=CARTESIAN_POINT('Origin',(0.,0.,0.));
#10462=CARTESIAN_POINT('',(1.24674050008925,0.,0.052360813993451));
#10463=CARTESIAN_POINT('Origin',(1.22833954473516,0.,0.));
#10464=CARTESIAN_POINT('Origin',(0.,0.,0.));
#10465=CARTESIAN_POINT('Origin',(0.,0.,0.));
#10466=CARTESIAN_POINT('',(-1.4,-0.1,1.71450551880629E-16));
#10467=CARTESIAN_POINT('Origin',(0.,-0.1,0.));
#10468=CARTESIAN_POINT('',(-1.4,0.,-1.71450551880629E-16));
#10469=CARTESIAN_POINT('Origin',(0.,-0.1,0.));
#10470=CARTESIAN_POINT('Origin',(0.,0.75,0.));
#10471=CARTESIAN_POINT('',(-1.4,0.75,1.71450551880629E-16));
#10472=CARTESIAN_POINT('Origin',(0.,0.75,0.));
#10473=CARTESIAN_POINT('',(1.22320001975977,0.75,0.246749348660852));
#10474=CARTESIAN_POINT('',(1.23958209161204,0.75,0.143317017690053));
#10475=CARTESIAN_POINT('Origin',(1.21321664662686,0.75,0.192154639568406));
#10476=CARTESIAN_POINT('',(1.24674050008925,0.75,0.052360813993448));
#10477=CARTESIAN_POINT('Origin',(0.,0.75,0.));
#10478=CARTESIAN_POINT('',(1.24674050008925,0.75,-0.052360813993448));
#10479=CARTESIAN_POINT('Origin',(1.22833954473516,0.75,0.));
#10480=CARTESIAN_POINT('',(1.23958209161204,0.75,-0.143317017690053));
#10481=CARTESIAN_POINT('Origin',(0.,0.75,0.));
#10482=CARTESIAN_POINT('',(1.22320001975977,0.75,-0.246749348660852));
#10483=CARTESIAN_POINT('Origin',(1.21321664662686,0.75,-0.192154639568406));
#10484=CARTESIAN_POINT('',(1.20190105810224,0.75,-0.335465908756113));
#10485=CARTESIAN_POINT('Origin',(0.,0.75,0.));
#10486=CARTESIAN_POINT('',(1.16954029537568,0.75,-0.435062095450087));
#10487=CARTESIAN_POINT('Origin',(1.1682203282434,0.75,-0.379577794185951));
#10488=CARTESIAN_POINT('',(1.13462523166105,0.75,-0.519354515801077));
#10489=CARTESIAN_POINT('Origin',(0.,0.75,0.));
#10490=CARTESIAN_POINT('',(1.08708260743774,0.75,-0.612662169561028));
#10491=CARTESIAN_POINT('Origin',(1.0944585482776,0.75,-0.557654483764164));
#10492=CARTESIAN_POINT('',(1.0394111664111,0.75,-0.690454891028201));
#10493=CARTESIAN_POINT('Origin',(0.,0.75,0.));
#10494=CARTESIAN_POINT('',(0.977857337884349,0.75,-0.775176467748211));
#10495=CARTESIAN_POINT('Origin',(0.993747566553533,0.75,-0.721999869202979));
#10496=CARTESIAN_POINT('',(0.918603348636233,0.75,-0.844553975349804));
#10497=CARTESIAN_POINT('Origin',(0.,0.75,0.));
#10498=CARTESIAN_POINT('',(0.844553975349804,0.75,-0.918603348636233));
#10499=CARTESIAN_POINT('Origin',(0.86856722168183,0.75,-0.86856722168183));
#10500=CARTESIAN_POINT('',(0.775176467748211,0.75,-0.977857337884349));
#10501=CARTESIAN_POINT('Origin',(0.,0.75,0.));
#10502=CARTESIAN_POINT('',(0.690454891028201,0.75,-1.0394111664111));
#10503=CARTESIAN_POINT('Origin',(0.721999869202979,0.75,-0.993747566553533));
#10504=CARTESIAN_POINT('',(0.612662169561028,0.75,-1.08708260743774));
#10505=CARTESIAN_POINT('Origin',(0.,0.75,0.));
#10506=CARTESIAN_POINT('',(0.519354515801077,0.75,-1.13462523166105));
#10507=CARTESIAN_POINT('Origin',(0.557654483764164,0.75,-1.0944585482776));
#10508=CARTESIAN_POINT('',(0.435062095450087,0.75,-1.16954029537568));
#10509=CARTESIAN_POINT('Origin',(0.,0.75,0.));
#10510=CARTESIAN_POINT('',(0.335465908756113,0.75,-1.20190105810224));
#10511=CARTESIAN_POINT('Origin',(0.379577794185951,0.75,-1.1682203282434));
#10512=CARTESIAN_POINT('',(0.246749348660852,0.75,-1.22320001975977));
#10513=CARTESIAN_POINT('Origin',(0.,0.75,0.));
#10514=CARTESIAN_POINT('',(0.143317017690053,0.75,-1.23958209161204));
#10515=CARTESIAN_POINT('Origin',(0.192154639568406,0.75,-1.21321664662686));
#10516=CARTESIAN_POINT('',(0.0523608139934481,0.75,-1.24674050008925));
#10517=CARTESIAN_POINT('Origin',(0.,0.75,0.));
#10518=CARTESIAN_POINT('',(-0.0523608139934479,0.75,-1.24674050008925));
#10519=CARTESIAN_POINT('Origin',(7.52141045863017E-17,0.75,-1.22833954473516));
#10520=CARTESIAN_POINT('',(-0.143317017690053,0.75,-1.23958209161204));
#10521=CARTESIAN_POINT('Origin',(0.,0.75,0.));
#10522=CARTESIAN_POINT('',(-0.246749348660852,0.75,-1.22320001975977));
#10523=CARTESIAN_POINT('Origin',(-0.192154639568406,0.75,-1.21321664662686));
#10524=CARTESIAN_POINT('',(-0.335465908756113,0.75,-1.20190105810224));
#10525=CARTESIAN_POINT('Origin',(0.,0.75,0.));
#10526=CARTESIAN_POINT('',(-0.435062095450087,0.75,-1.16954029537568));
#10527=CARTESIAN_POINT('Origin',(-0.379577794185951,0.75,-1.1682203282434));
#10528=CARTESIAN_POINT('',(-0.519354515801077,0.75,-1.13462523166105));
#10529=CARTESIAN_POINT('Origin',(0.,0.75,0.));
#10530=CARTESIAN_POINT('',(-0.612662169561028,0.75,-1.08708260743774));
#10531=CARTESIAN_POINT('Origin',(-0.557654483764164,0.75,-1.0944585482776));
#10532=CARTESIAN_POINT('',(-0.690454891028201,0.75,-1.0394111664111));
#10533=CARTESIAN_POINT('Origin',(0.,0.75,0.));
#10534=CARTESIAN_POINT('',(-0.775176467748211,0.75,-0.977857337884348));
#10535=CARTESIAN_POINT('Origin',(-0.721999869202979,0.75,-0.993747566553533));
#10536=CARTESIAN_POINT('',(-0.844553975349804,0.75,-0.918603348636233));
#10537=CARTESIAN_POINT('Origin',(0.,0.75,0.));
#10538=CARTESIAN_POINT('',(-0.918603348636233,0.75,-0.844553975349804));
#10539=CARTESIAN_POINT('Origin',(-0.86856722168183,0.75,-0.86856722168183));
#10540=CARTESIAN_POINT('',(-0.977857337884349,0.75,-0.775176467748211));
#10541=CARTESIAN_POINT('Origin',(0.,0.75,0.));
#10542=CARTESIAN_POINT('',(-1.0394111664111,0.75,-0.690454891028201));
#10543=CARTESIAN_POINT('Origin',(-0.993747566553533,0.75,-0.721999869202979));
#10544=CARTESIAN_POINT('',(-1.08708260743774,0.75,-0.612662169561029));
#10545=CARTESIAN_POINT('Origin',(0.,0.75,0.));
#10546=CARTESIAN_POINT('',(-1.13462523166105,0.75,-0.519354515801077));
#10547=CARTESIAN_POINT('Origin',(-1.0944585482776,0.75,-0.557654483764164));
#10548=CARTESIAN_POINT('',(-1.16954029537568,0.75,-0.435062095450087));
#10549=CARTESIAN_POINT('Origin',(0.,0.75,0.));
#10550=CARTESIAN_POINT('',(-1.20190105810224,0.75,-0.335465908756113));
#10551=CARTESIAN_POINT('Origin',(-1.1682203282434,0.75,-0.379577794185951));
#10552=CARTESIAN_POINT('',(-1.22320001975977,0.75,-0.246749348660852));
#10553=CARTESIAN_POINT('Origin',(0.,0.75,0.));
#10554=CARTESIAN_POINT('',(-1.23958209161204,0.75,-0.143317017690053));
#10555=CARTESIAN_POINT('Origin',(-1.21321664662686,0.75,-0.192154639568406));
#10556=CARTESIAN_POINT('',(-1.24674050008925,0.75,-0.0523608139934482));
#10557=CARTESIAN_POINT('Origin',(0.,0.75,0.));
#10558=CARTESIAN_POINT('',(-1.24674050008925,0.75,0.0523608139934479));
#10559=CARTESIAN_POINT('Origin',(-1.22833954473516,0.75,-1.50428209172603E-16));
#10560=CARTESIAN_POINT('',(-1.23958209161204,0.75,0.143317017690053));
#10561=CARTESIAN_POINT('Origin',(0.,0.75,0.));
#10562=CARTESIAN_POINT('',(-1.22320001975977,0.75,0.246749348660851));
#10563=CARTESIAN_POINT('Origin',(-1.21321664662686,0.75,0.192154639568406));
#10564=CARTESIAN_POINT('',(-1.20190105810224,0.75,0.335465908756113));
#10565=CARTESIAN_POINT('Origin',(0.,0.75,0.));
#10566=CARTESIAN_POINT('',(-1.16954029537568,0.75,0.435062095450087));
#10567=CARTESIAN_POINT('Origin',(-1.1682203282434,0.75,0.379577794185951));
#10568=CARTESIAN_POINT('',(-1.13462523166105,0.75,0.519354515801077));
#10569=CARTESIAN_POINT('Origin',(0.,0.75,0.));
#10570=CARTESIAN_POINT('',(-1.08708260743774,0.75,0.612662169561028));
#10571=CARTESIAN_POINT('Origin',(-1.0944585482776,0.75,0.557654483764164));
#10572=CARTESIAN_POINT('',(-1.0394111664111,0.75,0.690454891028201));
#10573=CARTESIAN_POINT('Origin',(0.,0.75,0.));
#10574=CARTESIAN_POINT('',(-0.977857337884348,0.75,0.775176467748211));
#10575=CARTESIAN_POINT('Origin',(-0.993747566553533,0.75,0.721999869202979));
#10576=CARTESIAN_POINT('',(-0.918603348636233,0.75,0.844553975349804));
#10577=CARTESIAN_POINT('Origin',(0.,0.75,0.));
#10578=CARTESIAN_POINT('',(-0.844553975349804,0.75,0.918603348636233));
#10579=CARTESIAN_POINT('Origin',(-0.86856722168183,0.75,0.86856722168183));
#10580=CARTESIAN_POINT('',(-0.775176467748211,0.75,0.977857337884349));
#10581=CARTESIAN_POINT('Origin',(0.,0.75,0.));
#10582=CARTESIAN_POINT('',(-0.690454891028201,0.75,1.0394111664111));
#10583=CARTESIAN_POINT('Origin',(-0.721999869202979,0.75,0.993747566553533));
#10584=CARTESIAN_POINT('',(-0.612662169561029,0.75,1.08708260743774));
#10585=CARTESIAN_POINT('Origin',(0.,0.75,0.));
#10586=CARTESIAN_POINT('',(-0.519354515801077,0.75,1.13462523166105));
#10587=CARTESIAN_POINT('Origin',(-0.557654483764164,0.75,1.0944585482776));
#10588=CARTESIAN_POINT('',(-0.435062095450087,0.75,1.16954029537568));
#10589=CARTESIAN_POINT('Origin',(0.,0.75,0.));
#10590=CARTESIAN_POINT('',(-0.335465908756113,0.75,1.20190105810224));
#10591=CARTESIAN_POINT('Origin',(-0.379577794185951,0.75,1.1682203282434));
#10592=CARTESIAN_POINT('',(-0.246749348660852,0.75,1.22320001975977));
#10593=CARTESIAN_POINT('Origin',(0.,0.75,0.));
#10594=CARTESIAN_POINT('',(-0.143317017690053,0.75,1.23958209161204));
#10595=CARTESIAN_POINT('Origin',(-0.192154639568406,0.75,1.21321664662686));
#10596=CARTESIAN_POINT('',(-0.0523608139934483,0.75,1.24674050008925));
#10597=CARTESIAN_POINT('Origin',(0.,0.75,0.));
#10598=CARTESIAN_POINT('',(0.0523608139934478,0.75,1.24674050008925));
#10599=CARTESIAN_POINT('Origin',(-2.25642313758905E-16,0.75,1.22833954473516));
#10600=CARTESIAN_POINT('',(0.143317017690053,0.75,1.23958209161204));
#10601=CARTESIAN_POINT('Origin',(0.,0.75,0.));
#10602=CARTESIAN_POINT('',(0.246749348660851,0.75,1.22320001975977));
#10603=CARTESIAN_POINT('Origin',(0.192154639568406,0.75,1.21321664662686));
#10604=CARTESIAN_POINT('',(0.335465908756113,0.75,1.20190105810224));
#10605=CARTESIAN_POINT('Origin',(0.,0.75,0.));
#10606=CARTESIAN_POINT('',(0.435062095450087,0.75,1.16954029537568));
#10607=CARTESIAN_POINT('Origin',(0.379577794185951,0.75,1.1682203282434));
#10608=CARTESIAN_POINT('',(0.519354515801077,0.75,1.13462523166105));
#10609=CARTESIAN_POINT('Origin',(0.,0.75,0.));
#10610=CARTESIAN_POINT('',(0.612662169561028,0.75,1.08708260743774));
#10611=CARTESIAN_POINT('Origin',(0.557654483764164,0.75,1.0944585482776));
#10612=CARTESIAN_POINT('',(0.690454891028201,0.75,1.0394111664111));
#10613=CARTESIAN_POINT('Origin',(0.,0.75,0.));
#10614=CARTESIAN_POINT('',(0.775176467748211,0.75,0.977857337884349));
#10615=CARTESIAN_POINT('Origin',(0.721999869202979,0.75,0.993747566553533));
#10616=CARTESIAN_POINT('',(0.844553975349804,0.75,0.918603348636233));
#10617=CARTESIAN_POINT('Origin',(0.,0.75,0.));
#10618=CARTESIAN_POINT('',(0.918603348636233,0.75,0.844553975349804));
#10619=CARTESIAN_POINT('Origin',(0.86856722168183,0.75,0.86856722168183));
#10620=CARTESIAN_POINT('',(0.977857337884349,0.75,0.775176467748211));
#10621=CARTESIAN_POINT('Origin',(0.,0.75,0.));
#10622=CARTESIAN_POINT('',(1.0394111664111,0.75,0.690454891028201));
#10623=CARTESIAN_POINT('Origin',(0.993747566553533,0.75,0.72199986920298));
#10624=CARTESIAN_POINT('',(1.08708260743774,0.75,0.612662169561029));
#10625=CARTESIAN_POINT('Origin',(0.,0.75,0.));
#10626=CARTESIAN_POINT('',(1.13462523166105,0.75,0.519354515801077));
#10627=CARTESIAN_POINT('Origin',(1.0944585482776,0.75,0.557654483764164));
#10628=CARTESIAN_POINT('',(1.16954029537568,0.75,0.435062095450087));
#10629=CARTESIAN_POINT('Origin',(0.,0.75,0.));
#10630=CARTESIAN_POINT('',(1.20190105810224,0.75,0.335465908756113));
#10631=CARTESIAN_POINT('Origin',(1.1682203282434,0.75,0.379577794185952));
#10632=CARTESIAN_POINT('Origin',(0.,0.75,0.));
#10633=CARTESIAN_POINT('Origin',(0.,0.75,0.));
#10634=CARTESIAN_POINT('',(-1.4,0.75,1.71450551880629E-16));
#10635=CARTESIAN_POINT('Origin',(1.21321664662686,0.,0.192154639568406));
#10636=CARTESIAN_POINT('',(1.23958209161204,0.,0.14331701769005));
#10637=CARTESIAN_POINT('',(1.22320001975977,0.,0.246749348660855));
#10638=CARTESIAN_POINT('Origin',(0.,0.,0.));
#10639=CARTESIAN_POINT('',(1.20190105810224,0.,0.33546590875611));
#10640=CARTESIAN_POINT('Origin',(1.1682203282434,0.,0.379577794185952));
#10641=CARTESIAN_POINT('',(1.16954029537568,0.,0.43506209545009));
#10642=CARTESIAN_POINT('Origin',(0.,0.,0.));
#10643=CARTESIAN_POINT('',(1.13462523166105,0.,0.519354515801074));
#10644=CARTESIAN_POINT('Origin',(1.0944585482776,0.,0.557654483764164));
#10645=CARTESIAN_POINT('',(1.08708260743774,0.,0.612662169561031));
#10646=CARTESIAN_POINT('Origin',(0.,0.,0.));
#10647=CARTESIAN_POINT('',(1.03941116641111,0.,0.690454891028199));
#10648=CARTESIAN_POINT('Origin',(0.993747566553533,0.,0.72199986920298));
#10649=CARTESIAN_POINT('',(0.977857337884347,0.,0.775176467748214));
#10650=CARTESIAN_POINT('Origin',(0.,0.,0.));
#10651=CARTESIAN_POINT('',(0.918603348636235,0.,0.844553975349802));
#10652=CARTESIAN_POINT('Origin',(0.86856722168183,0.,0.86856722168183));
#10653=CARTESIAN_POINT('',(0.844553975349802,0.,0.918603348636235));
#10654=CARTESIAN_POINT('Origin',(0.,0.,0.));
#10655=CARTESIAN_POINT('',(0.775176467748213,0.,0.977857337884347));
#10656=CARTESIAN_POINT('Origin',(0.721999869202979,0.,0.993747566553533));
#10657=CARTESIAN_POINT('',(0.690454891028198,0.,1.03941116641111));
#10658=CARTESIAN_POINT('Origin',(0.,0.,0.));
#10659=CARTESIAN_POINT('',(0.612662169561031,0.,1.08708260743774));
#10660=CARTESIAN_POINT('Origin',(0.557654483764164,0.,1.0944585482776));
#10661=CARTESIAN_POINT('',(0.519354515801074,0.,1.13462523166105));
#10662=CARTESIAN_POINT('Origin',(0.,0.,0.));
#10663=CARTESIAN_POINT('',(0.43506209545009,0.,1.16954029537568));
#10664=CARTESIAN_POINT('Origin',(0.379577794185951,0.,1.1682203282434));
#10665=CARTESIAN_POINT('',(0.33546590875611,0.,1.20190105810224));
#10666=CARTESIAN_POINT('Origin',(0.,0.,0.));
#10667=CARTESIAN_POINT('',(0.246749348660854,0.,1.22320001975977));
#10668=CARTESIAN_POINT('Origin',(0.192154639568406,0.,1.21321664662686));
#10669=CARTESIAN_POINT('',(0.14331701769005,0.,1.23958209161204));
#10670=CARTESIAN_POINT('Origin',(0.,0.,0.));
#10671=CARTESIAN_POINT('',(0.0523608139934508,0.,1.24674050008925));
#10672=CARTESIAN_POINT('Origin',(-2.25642313758905E-16,0.,1.22833954473516));
#10673=CARTESIAN_POINT('',(-0.0523608139934513,0.,1.24674050008925));
#10674=CARTESIAN_POINT('Origin',(0.,0.,0.));
#10675=CARTESIAN_POINT('',(-0.14331701769005,0.,1.23958209161204));
#10676=CARTESIAN_POINT('Origin',(-0.192154639568406,0.,1.21321664662686));
#10677=CARTESIAN_POINT('',(-0.246749348660855,0.,1.22320001975977));
#10678=CARTESIAN_POINT('Origin',(0.,0.,0.));
#10679=CARTESIAN_POINT('',(-0.33546590875611,0.,1.20190105810224));
#10680=CARTESIAN_POINT('Origin',(-0.379577794185951,0.,1.1682203282434));
#10681=CARTESIAN_POINT('',(-0.43506209545009,0.,1.16954029537568));
#10682=CARTESIAN_POINT('Origin',(0.,0.,0.));
#10683=CARTESIAN_POINT('',(-0.519354515801074,0.,1.13462523166105));
#10684=CARTESIAN_POINT('Origin',(-0.557654483764164,0.,1.0944585482776));
#10685=CARTESIAN_POINT('',(-0.612662169561031,0.,1.08708260743774));
#10686=CARTESIAN_POINT('Origin',(0.,0.,0.));
#10687=CARTESIAN_POINT('',(-0.690454891028199,0.,1.03941116641111));
#10688=CARTESIAN_POINT('Origin',(-0.721999869202979,0.,0.993747566553533));
#10689=CARTESIAN_POINT('',(-0.775176467748213,0.,0.977857337884347));
#10690=CARTESIAN_POINT('Origin',(0.,0.,0.));
#10691=CARTESIAN_POINT('',(-0.844553975349802,0.,0.918603348636235));
#10692=CARTESIAN_POINT('Origin',(-0.86856722168183,0.,0.86856722168183));
#10693=CARTESIAN_POINT('',(-0.918603348636235,0.,0.844553975349802));
#10694=CARTESIAN_POINT('Origin',(0.,0.,0.));
#10695=CARTESIAN_POINT('',(-0.977857337884347,0.,0.775176467748213));
#10696=CARTESIAN_POINT('Origin',(-0.993747566553533,0.,0.721999869202979));
#10697=CARTESIAN_POINT('',(-1.03941116641111,0.,0.690454891028198));
#10698=CARTESIAN_POINT('Origin',(0.,0.,0.));
#10699=CARTESIAN_POINT('',(-1.08708260743774,0.,0.612662169561031));
#10700=CARTESIAN_POINT('Origin',(-1.0944585482776,0.,0.557654483764164));
#10701=CARTESIAN_POINT('',(-1.13462523166105,0.,0.519354515801074));
#10702=CARTESIAN_POINT('Origin',(0.,0.,0.));
#10703=CARTESIAN_POINT('',(-1.16954029537568,0.,0.43506209545009));
#10704=CARTESIAN_POINT('Origin',(-1.1682203282434,0.,0.379577794185951));
#10705=CARTESIAN_POINT('',(-1.20190105810224,0.,0.33546590875611));
#10706=CARTESIAN_POINT('Origin',(0.,0.,0.));
#10707=CARTESIAN_POINT('',(-1.22320001975977,0.,0.246749348660854));
#10708=CARTESIAN_POINT('Origin',(-1.21321664662686,0.,0.192154639568406));
#10709=CARTESIAN_POINT('',(-1.23958209161204,0.,0.14331701769005));
#10710=CARTESIAN_POINT('Origin',(0.,0.,0.));
#10711=CARTESIAN_POINT('',(-1.24674050008925,0.,0.0523608139934509));
#10712=CARTESIAN_POINT('Origin',(-1.22833954473516,0.,-1.50428209172603E-16));
#10713=CARTESIAN_POINT('',(-1.24674050008925,0.,-0.0523608139934512));
#10714=CARTESIAN_POINT('Origin',(0.,0.,0.));
#10715=CARTESIAN_POINT('',(-1.23958209161204,0.,-0.14331701769005));
#10716=CARTESIAN_POINT('Origin',(-1.21321664662686,0.,-0.192154639568406));
#10717=CARTESIAN_POINT('',(-1.22320001975977,0.,-0.246749348660855));
#10718=CARTESIAN_POINT('Origin',(0.,0.,0.));
#10719=CARTESIAN_POINT('',(-1.20190105810224,0.,-0.33546590875611));
#10720=CARTESIAN_POINT('Origin',(-1.1682203282434,0.,-0.379577794185951));
#10721=CARTESIAN_POINT('',(-1.16954029537568,0.,-0.43506209545009));
#10722=CARTESIAN_POINT('Origin',(0.,0.,0.));
#10723=CARTESIAN_POINT('',(-1.13462523166105,0.,-0.519354515801074));
#10724=CARTESIAN_POINT('Origin',(-1.0944585482776,0.,-0.557654483764164));
#10725=CARTESIAN_POINT('',(-1.08708260743774,0.,-0.612662169561031));
#10726=CARTESIAN_POINT('Origin',(0.,0.,0.));
#10727=CARTESIAN_POINT('',(-1.03941116641111,0.,-0.690454891028199));
#10728=CARTESIAN_POINT('Origin',(-0.993747566553533,0.,-0.721999869202979));
#10729=CARTESIAN_POINT('',(-0.977857337884347,0.,-0.775176467748213));
#10730=CARTESIAN_POINT('Origin',(0.,0.,0.));
#10731=CARTESIAN_POINT('',(-0.918603348636235,0.,-0.844553975349802));
#10732=CARTESIAN_POINT('Origin',(-0.86856722168183,0.,-0.86856722168183));
#10733=CARTESIAN_POINT('',(-0.844553975349802,0.,-0.918603348636235));
#10734=CARTESIAN_POINT('Origin',(0.,0.,0.));
#10735=CARTESIAN_POINT('',(-0.775176467748213,0.,-0.977857337884347));
#10736=CARTESIAN_POINT('Origin',(-0.721999869202979,0.,-0.993747566553533));
#10737=CARTESIAN_POINT('',(-0.690454891028198,0.,-1.03941116641111));
#10738=CARTESIAN_POINT('Origin',(0.,0.,0.));
#10739=CARTESIAN_POINT('',(-0.612662169561031,0.,-1.08708260743774));
#10740=CARTESIAN_POINT('Origin',(-0.557654483764164,0.,-1.0944585482776));
#10741=CARTESIAN_POINT('',(-0.519354515801074,0.,-1.13462523166105));
#10742=CARTESIAN_POINT('Origin',(0.,0.,0.));
#10743=CARTESIAN_POINT('',(-0.43506209545009,0.,-1.16954029537568));
#10744=CARTESIAN_POINT('Origin',(-0.379577794185951,0.,-1.1682203282434));
#10745=CARTESIAN_POINT('',(-0.33546590875611,0.,-1.20190105810224));
#10746=CARTESIAN_POINT('Origin',(0.,0.,0.));
#10747=CARTESIAN_POINT('',(-0.246749348660854,0.,-1.22320001975977));
#10748=CARTESIAN_POINT('Origin',(-0.192154639568406,0.,-1.21321664662686));
#10749=CARTESIAN_POINT('',(-0.14331701769005,0.,-1.23958209161204));
#10750=CARTESIAN_POINT('Origin',(0.,0.,0.));
#10751=CARTESIAN_POINT('',(-0.052360813993451,0.,-1.24674050008925));
#10752=CARTESIAN_POINT('Origin',(7.52141045863017E-17,0.,-1.22833954473516));
#10753=CARTESIAN_POINT('',(0.0523608139934511,0.,-1.24674050008925));
#10754=CARTESIAN_POINT('Origin',(0.,0.,0.));
#10755=CARTESIAN_POINT('',(0.14331701769005,0.,-1.23958209161204));
#10756=CARTESIAN_POINT('Origin',(0.192154639568406,0.,-1.21321664662686));
#10757=CARTESIAN_POINT('',(0.246749348660855,0.,-1.22320001975977));
#10758=CARTESIAN_POINT('Origin',(0.,0.,0.));
#10759=CARTESIAN_POINT('',(0.33546590875611,0.,-1.20190105810224));
#10760=CARTESIAN_POINT('Origin',(0.379577794185951,0.,-1.1682203282434));
#10761=CARTESIAN_POINT('',(0.43506209545009,0.,-1.16954029537568));
#10762=CARTESIAN_POINT('Origin',(0.,0.,0.));
#10763=CARTESIAN_POINT('',(0.519354515801074,0.,-1.13462523166105));
#10764=CARTESIAN_POINT('Origin',(0.557654483764164,0.,-1.0944585482776));
#10765=CARTESIAN_POINT('',(0.612662169561031,0.,-1.08708260743774));
#10766=CARTESIAN_POINT('Origin',(0.,0.,0.));
#10767=CARTESIAN_POINT('',(0.690454891028198,0.,-1.03941116641111));
#10768=CARTESIAN_POINT('Origin',(0.721999869202979,0.,-0.993747566553533));
#10769=CARTESIAN_POINT('',(0.775176467748213,0.,-0.977857337884347));
#10770=CARTESIAN_POINT('Origin',(0.,0.,0.));
#10771=CARTESIAN_POINT('',(0.844553975349802,0.,-0.918603348636235));
#10772=CARTESIAN_POINT('Origin',(0.86856722168183,0.,-0.86856722168183));
#10773=CARTESIAN_POINT('',(0.918603348636235,0.,-0.844553975349802));
#10774=CARTESIAN_POINT('Origin',(0.,0.,0.));
#10775=CARTESIAN_POINT('',(0.977857337884347,0.,-0.775176467748213));
#10776=CARTESIAN_POINT('Origin',(0.993747566553533,0.,-0.721999869202979));
#10777=CARTESIAN_POINT('',(1.03941116641111,0.,-0.690454891028198));
#10778=CARTESIAN_POINT('Origin',(0.,0.,0.));
#10779=CARTESIAN_POINT('',(1.08708260743774,0.,-0.612662169561031));
#10780=CARTESIAN_POINT('Origin',(1.0944585482776,0.,-0.557654483764164));
#10781=CARTESIAN_POINT('',(1.13462523166105,0.,-0.519354515801074));
#10782=CARTESIAN_POINT('Origin',(0.,0.,0.));
#10783=CARTESIAN_POINT('',(1.16954029537568,0.,-0.43506209545009));
#10784=CARTESIAN_POINT('Origin',(1.1682203282434,0.,-0.379577794185951));
#10785=CARTESIAN_POINT('',(1.20190105810224,0.,-0.33546590875611));
#10786=CARTESIAN_POINT('Origin',(0.,0.,0.));
#10787=CARTESIAN_POINT('',(1.22320001975977,0.,-0.246749348660855));
#10788=CARTESIAN_POINT('Origin',(1.21321664662686,0.,-0.192154639568406));
#10789=CARTESIAN_POINT('',(1.23958209161204,0.,-0.14331701769005));
#10790=CARTESIAN_POINT('Origin',(0.,0.,0.));
#10791=CARTESIAN_POINT('',(1.24674050008925,0.,0.052360813993451));
#10792=CARTESIAN_POINT('Origin',(1.22833954473516,0.,0.));
#10793=CARTESIAN_POINT('',(1.24674050008925,0.,-0.052360813993451));
#10794=CARTESIAN_POINT('Origin',(0.,0.,0.));
#10933=UNCERTAINTY_MEASURE_WITH_UNIT(LENGTH_MEASURE(0.001),#10964,
'DISTANCE_ACCURACY_VALUE',
'Maximum model space distance between geometric entities at asserted c
onnectivities');
#10936=UNCERTAINTY_MEASURE_WITH_UNIT(LENGTH_MEASURE(0.001),#10964,
'DISTANCE_ACCURACY_VALUE',
'Maximum model space distance between geometric entities at asserted c
onnectivities');
#10960=(
GEOMETRIC_REPRESENTATION_CONTEXT(3)
GLOBAL_UNCERTAINTY_ASSIGNED_CONTEXT((#10933))
GLOBAL_UNIT_ASSIGNED_CONTEXT((#10964,#10966,#10967))
REPRESENTATION_CONTEXT('','3D')
);
#10963=(
GEOMETRIC_REPRESENTATION_CONTEXT(3)
GLOBAL_UNCERTAINTY_ASSIGNED_CONTEXT((#10936))
GLOBAL_UNIT_ASSIGNED_CONTEXT((#10964,#10966,#10967))
REPRESENTATION_CONTEXT('','3D')
);
#10964=(
LENGTH_UNIT()
NAMED_UNIT(*)
SI_UNIT(.CENTI.,.METRE.)
);
#10966=(
NAMED_UNIT(*)
PLANE_ANGLE_UNIT()
SI_UNIT($,.RADIAN.)
);
#10967=(
NAMED_UNIT(*)
SI_UNIT($,.STERADIAN.)
SOLID_ANGLE_UNIT()
);
#10991=SHAPE_DEFINITION_REPRESENTATION(#11044,#11080);
#11044=PRODUCT_DEFINITION_SHAPE('',$,#11107);
#11080=SHAPE_REPRESENTATION('',(#6384),#10960);
#11083=PRODUCT_DEFINITION_CONTEXT('part definition',#11163,'design');
#11107=PRODUCT_DEFINITION(
'Timing Pulley - 2 mm Pitch, 40 Teeth, 12 mm Bore',
'Timing Pulley - 2 mm Pitch, 40 Teeth, 12 mm Bore',#11133,#11083);
#11133=PRODUCT_DEFINITION_FORMATION('',$,#11188);
#11163=APPLICATION_CONTEXT(
'Core Data for Automotive Mechanical Design Process');
#11164=PRODUCT_CONTEXT('part definition',#11163,'mechanical');
#11188=PRODUCT('Timing Pulley - 2 mm Pitch, 40 Teeth, 12 mm Bore',
'Timing Pulley - 2 mm Pitch, 40 Teeth, 12 mm Bore',
'Timing Pulley - 2 mm Pitch, 40 Teeth, 12 mm Bore',(#11164));
#11240=COLOUR_RGB('Sky Blue',0.24,0.69,0.87);
#11241=FILL_AREA_STYLE_COLOUR('',#11240);
#11242=FILL_AREA_STYLE('',(#11241));
#11243=SURFACE_STYLE_FILL_AREA(#11242);
#11244=SURFACE_SIDE_STYLE('',(#11243));
#11245=SURFACE_STYLE_USAGE(.BOTH.,#11244);
#11246=PRESENTATION_STYLE_ASSIGNMENT((#11245));
ENDSEC;
END-ISO-10303-21;
